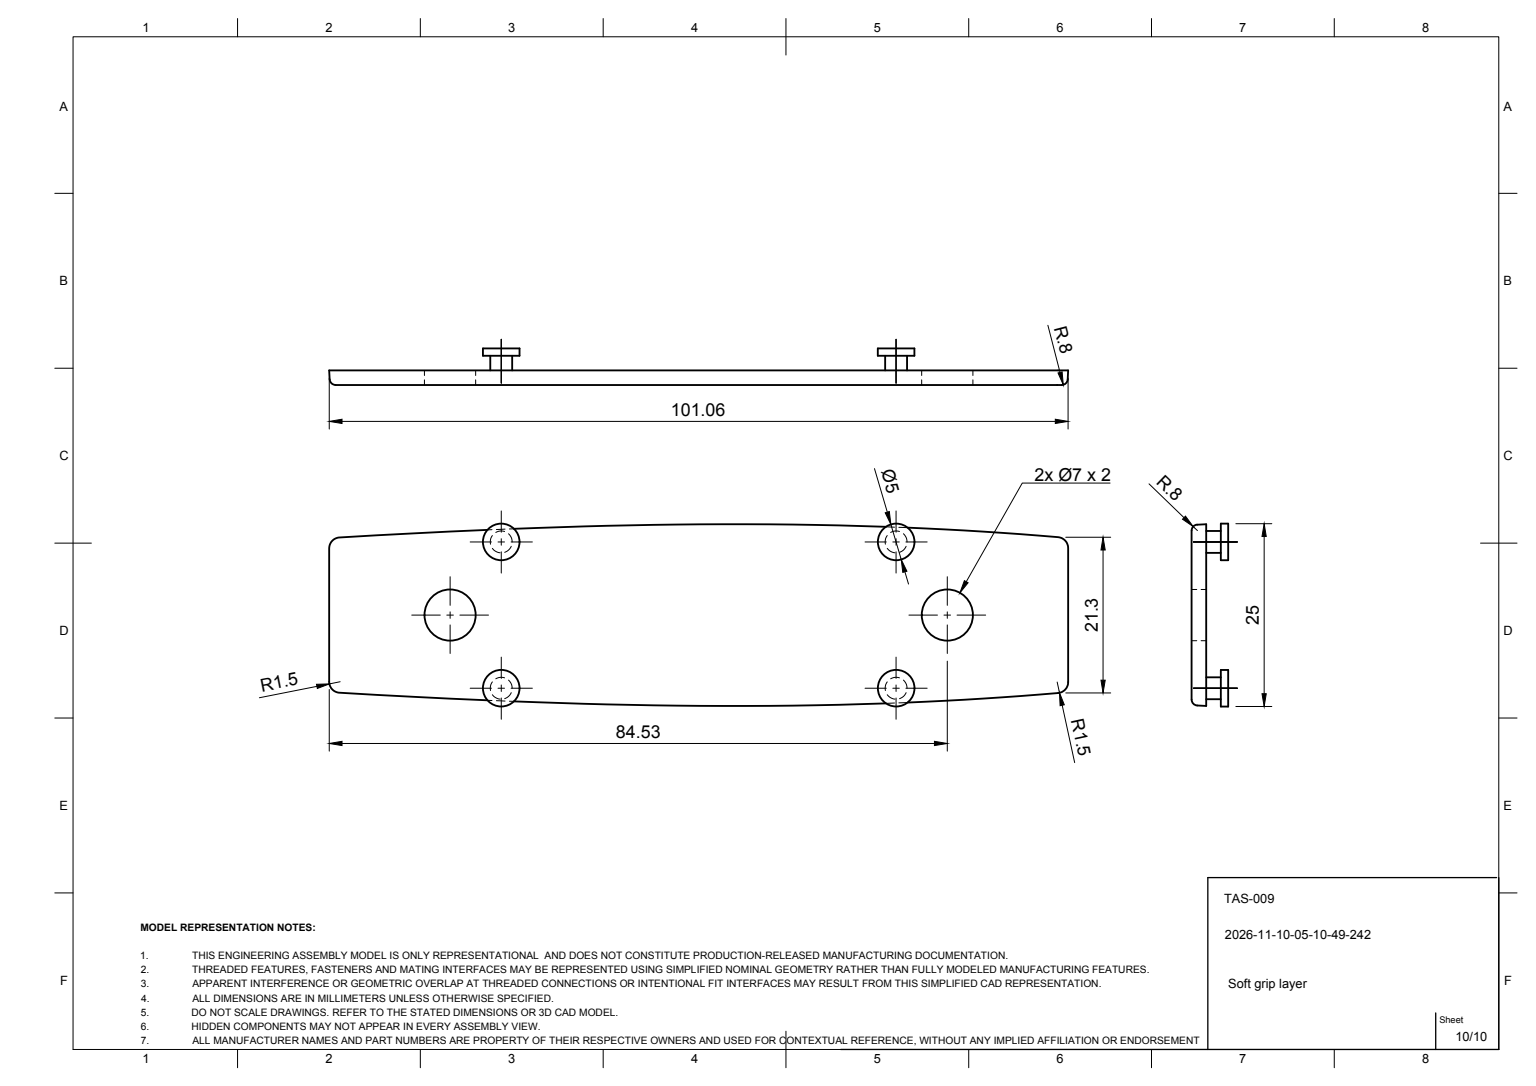
ISO-10303-21;
HEADER;
/* Generated by software containing ST-Developer
 * from STEP Tools, Inc. (www.steptools.com) 
 */

FILE_DESCRIPTION(
/* description */ (''),
/* implementation_level */ '2;1');

FILE_NAME(
/* name */ 'Soft grip layer.step',
/* time_stamp */ '2026-11-12T00:53:40-08:00',
/* author */ (''),
/* organization */ (''),
/* preprocessor_version */ 'ST-DEVELOPER v20.2',
/* originating_system */ 'Autodesk Translation Framework v15.17.0.0',
/* authorisation */ '');

FILE_SCHEMA (('AUTOMOTIVE_DESIGN { 1 0 10303 214 3 1 1 }'));
ENDSEC;

DATA;
#10=MECHANICAL_DESIGN_GEOMETRIC_PRESENTATION_REPRESENTATION('',(#579),#22129);
#160=B_SPLINE_SURFACE_WITH_KNOTS('',3,3,((#21557,#21558,#21559,#21560,#21561),
(#21562,#21563,#21564,#21565,#21566),(#21567,#21568,#21569,#21570,#21571),
(#21572,#21573,#21574,#21575,#21576),(#21577,#21578,#21579,#21580,#21581)),
 .UNSPECIFIED.,.F.,.F.,.F.,(4,1,4),(4,1,4),(0.,0.571428571428571,1.),(0.,
0.0453052401185593,0.105712226943305),.UNSPECIFIED.);
#161=B_SPLINE_SURFACE_WITH_KNOTS('',3,3,((#21604,#21605,#21606,#21607,#21608),
(#21609,#21610,#21611,#21612,#21613),(#21614,#21615,#21616,#21617,#21618),
(#21619,#21620,#21621,#21622,#21623),(#21624,#21625,#21626,#21627,#21628)),
 .UNSPECIFIED.,.F.,.F.,.F.,(4,1,4),(4,1,4),(0.,0.571428571428571,1.),(0.,
0.0453052401439183,0.105712227002476),.UNSPECIFIED.);
#162=B_SPLINE_SURFACE_WITH_KNOTS('',3,3,((#21642,#21643,#21644,#21645,#21646),
(#21647,#21648,#21649,#21650,#21651),(#21652,#21653,#21654,#21655,#21656),
(#21657,#21658,#21659,#21660,#21661),(#21662,#21663,#21664,#21665,#21666)),
 .UNSPECIFIED.,.F.,.F.,.F.,(4,1,4),(4,1,4),(0.,0.571428571428571,1.),(0.,
4.20509945658767,9.8118987320379),.UNSPECIFIED.);
#163=B_SPLINE_SURFACE_WITH_KNOTS('',3,3,((#21680,#21681,#21682,#21683,#21684),
(#21685,#21686,#21687,#21688,#21689),(#21690,#21691,#21692,#21693,#21694),
(#21695,#21696,#21697,#21698,#21699),(#21700,#21701,#21702,#21703,#21704)),
 .UNSPECIFIED.,.F.,.F.,.F.,(4,1,4),(4,1,4),(0.,0.571428571428571,1.),(0.,
0.0444882141544403,0.103805833027027),.UNSPECIFIED.);
#164=B_SPLINE_SURFACE_WITH_KNOTS('',3,3,((#21724,#21725,#21726,#21727,#21728),
(#21729,#21730,#21731,#21732,#21733),(#21734,#21735,#21736,#21737,#21738),
(#21739,#21740,#21741,#21742,#21743),(#21744,#21745,#21746,#21747,#21748)),
 .UNSPECIFIED.,.F.,.F.,.F.,(4,1,4),(4,1,4),(0.,0.571428571428571,1.),(2.06005858395869E-18,
0.0444882141931362,0.103805833117318),.UNSPECIFIED.);
#165=B_SPLINE_SURFACE_WITH_KNOTS('',3,3,((#21762,#21763,#21764,#21765,#21766),
(#21767,#21768,#21769,#21770,#21771),(#21772,#21773,#21774,#21775,#21776),
(#21777,#21778,#21779,#21780,#21781),(#21782,#21783,#21784,#21785,#21786)),
 .UNSPECIFIED.,.F.,.F.,.F.,(4,1,4),(4,1,4),(0.,0.571428571428571,1.),(0.,
4.20509909783593,9.81189789495051),.UNSPECIFIED.);
#166=B_SPLINE_SURFACE_WITH_KNOTS('',3,3,((#21809,#21810,#21811,#21812),
(#21813,#21814,#21815,#21816),(#21817,#21818,#21819,#21820),(#21821,#21822,
#21823,#21824),(#21825,#21826,#21827,#21828)),.UNSPECIFIED.,.F.,.F.,.F.,
(4,1,4),(4,4),(0.,0.571428571428571,1.),(-0.00268702576369722,0.125151053668407),
 .UNSPECIFIED.);
#167=B_SPLINE_SURFACE_WITH_KNOTS('',3,3,((#21862,#21863,#21864,#21865),
(#21866,#21867,#21868,#21869),(#21870,#21871,#21872,#21873),(#21874,#21875,
#21876,#21877)),.UNSPECIFIED.,.F.,.F.,.F.,(4,4),(4,4),(0.0135518988075539,
0.986045335056424),(0.,0.622596671418298),.UNSPECIFIED.);
#168=B_SPLINE_SURFACE_WITH_KNOTS('',3,3,((#21887,#21888,#21889,#21890),
(#21891,#21892,#21893,#21894),(#21895,#21896,#21897,#21898),(#21899,#21900,
#21901,#21902),(#21903,#21904,#21905,#21906)),.UNSPECIFIED.,.F.,.F.,.F.,
(4,1,4),(4,4),(0.,0.571428571428571,1.),(-0.00281084541253883,0.124959300034279),
 .UNSPECIFIED.);
#169=B_SPLINE_SURFACE_WITH_KNOTS('',3,3,((#21948,#21949,#21950,#21951),
(#21952,#21953,#21954,#21955),(#21956,#21957,#21958,#21959),(#21960,#21961,
#21962,#21963),(#21964,#21965,#21966,#21967)),.UNSPECIFIED.,.F.,.F.,.F.,
(4,1,4),(4,4),(0.,0.571428571428571,1.),(-0.00261432509268751,0.125151053668407),
 .UNSPECIFIED.);
#170=B_SPLINE_SURFACE_WITH_KNOTS('',3,3,((#22001,#22002,#22003,#22004),
(#22005,#22006,#22007,#22008),(#22009,#22010,#22011,#22012),(#22013,#22014,
#22015,#22016),(#22017,#22018,#22019,#22020)),.UNSPECIFIED.,.F.,.F.,.F.,
(4,1,4),(4,4),(0.,0.571428571428571,1.),(-0.00286362952972032,0.12495930003428),
 .UNSPECIFIED.);
#171=B_SPLINE_SURFACE_WITH_KNOTS('',3,3,((#22059,#22060,#22061,#22062),
(#22063,#22064,#22065,#22066),(#22067,#22068,#22069,#22070),(#22071,#22072,
#22073,#22074)),.UNSPECIFIED.,.F.,.F.,.F.,(4,4),(4,4),(0.0139546649435754,
0.986448101192446),(0.,0.622596671418299),.UNSPECIFIED.);
#528=B_SPLINE_CURVE_WITH_KNOTS('',3,(#21586,#21587,#21588,#21589,#21590),
 .UNSPECIFIED.,.F.,.F.,(4,1,4),(-0.105712226943305,-0.0453052401185593,
0.),.UNSPECIFIED.);
#529=B_SPLINE_CURVE_WITH_KNOTS('',3,(#21593,#21594,#21595,#21596,#21597),
 .UNSPECIFIED.,.F.,.F.,(4,1,4),(0.,0.0453052401185593,0.105712226943305),
 .UNSPECIFIED.);
#530=B_SPLINE_CURVE_WITH_KNOTS('',3,(#21632,#21633,#21634,#21635,#21636),
 .UNSPECIFIED.,.F.,.F.,(4,1,4),(-0.105712227002476,-0.0453052401439183,
0.),.UNSPECIFIED.);
#531=B_SPLINE_CURVE_WITH_KNOTS('',3,(#21637,#21638,#21639,#21640,#21641),
 .UNSPECIFIED.,.F.,.F.,(4,1,4),(0.,0.0453052401439183,0.105712227002476),
 .UNSPECIFIED.);
#532=B_SPLINE_CURVE_WITH_KNOTS('',3,(#21670,#21671,#21672,#21673,#21674),
 .UNSPECIFIED.,.F.,.F.,(4,1,4),(-9.8118987320379,-4.20509945658767,0.),
 .UNSPECIFIED.);
#533=B_SPLINE_CURVE_WITH_KNOTS('',3,(#21675,#21676,#21677,#21678,#21679),
 .UNSPECIFIED.,.F.,.F.,(4,1,4),(0.,4.20509945658767,9.8118987320379),
 .UNSPECIFIED.);
#534=B_SPLINE_CURVE_WITH_KNOTS('',3,(#21708,#21709,#21710,#21711,#21712),
 .UNSPECIFIED.,.F.,.F.,(4,1,4),(-0.103805833027027,-0.0444882141544403,
0.),.UNSPECIFIED.);
#535=B_SPLINE_CURVE_WITH_KNOTS('',3,(#21713,#21714,#21715,#21716,#21717),
 .UNSPECIFIED.,.F.,.F.,(4,1,4),(0.,0.0444882141544403,0.103805833027027),
 .UNSPECIFIED.);
#536=B_SPLINE_CURVE_WITH_KNOTS('',3,(#21752,#21753,#21754,#21755,#21756),
 .UNSPECIFIED.,.F.,.F.,(4,1,4),(-0.103805833117318,-0.0444882141931362,
-2.06005858395869E-18),.UNSPECIFIED.);
#537=B_SPLINE_CURVE_WITH_KNOTS('',3,(#21757,#21758,#21759,#21760,#21761),
 .UNSPECIFIED.,.F.,.F.,(4,1,4),(2.06005858395869E-18,0.0444882141931362,
0.103805833117318),.UNSPECIFIED.);
#538=B_SPLINE_CURVE_WITH_KNOTS('',3,(#21787,#21788,#21789,#21790,#21791),
 .UNSPECIFIED.,.F.,.F.,(4,1,4),(-9.81189789495051,-4.20509909783593,0.),
 .UNSPECIFIED.);
#539=B_SPLINE_CURVE_WITH_KNOTS('',3,(#21792,#21793,#21794,#21795,#21796),
 .UNSPECIFIED.,.F.,.F.,(4,1,4),(0.,4.20509909783593,9.81189789495051),
 .UNSPECIFIED.);
#540=B_SPLINE_CURVE_WITH_KNOTS('',3,(#21799,#21800,#21801,#21802),
 .UNSPECIFIED.,.F.,.F.,(4,4),(0.00062434729305816,0.125151053668407),
 .UNSPECIFIED.);
#541=B_SPLINE_CURVE_WITH_KNOTS('',3,(#21805,#21806,#21807,#21808),
 .UNSPECIFIED.,.F.,.F.,(4,4),(-0.125151053668407,-0.000624347293058304),
 .UNSPECIFIED.);
#542=B_SPLINE_CURVE_WITH_KNOTS('',3,(#21830,#21831,#21832,#21833),
 .UNSPECIFIED.,.F.,.F.,(4,4),(-0.124859357077656,3.91613824701764E-16),
 .UNSPECIFIED.);
#543=B_SPLINE_CURVE_WITH_KNOTS('',3,(#21834,#21835,#21836,#21837,#21838,
#21839,#21840,#21841,#21842,#21843,#21844,#21845,#21846,#21847,#21848,#21849,
#21850,#21851,#21852,#21853,#21854,#21855,#21856,#21857,#21858,#21859,#21860,
#21861),.UNSPECIFIED.,.F.,.F.,(4,3,3,3,3,3,3,3,3,4),(0.,0.032270992282214,
0.0586131010579366,0.0908535483049998,0.095660418056781,0.117090121226367,
0.149479430319939,0.17008966569926,0.202270498561131,0.223122165115773),
 .UNSPECIFIED.);
#544=B_SPLINE_CURVE_WITH_KNOTS('',3,(#21879,#21880,#21881,#21882),
 .UNSPECIFIED.,.F.,.F.,(4,4),(1.57426155444895E-16,0.124757292074316),
 .UNSPECIFIED.);
#545=B_SPLINE_CURVE_WITH_KNOTS('',3,(#21883,#21884,#21885,#21886),
 .UNSPECIFIED.,.F.,.F.,(4,4),(0.0135518988075539,0.986045335056425),
 .UNSPECIFIED.);
#546=B_SPLINE_CURVE_WITH_KNOTS('',3,(#21908,#21909,#21910,#21911),
 .UNSPECIFIED.,.F.,.F.,(4,4),(-0.124959300034279,-0.000432357919845506),
 .UNSPECIFIED.);
#547=B_SPLINE_CURVE_WITH_KNOTS('',3,(#21912,#21913,#21914,#21915,#21916,
#21917,#21918,#21919,#21920,#21921,#21922,#21923,#21924,#21925,#21926,#21927,
#21928,#21929,#21930,#21931,#21932,#21933,#21934,#21935,#21936,#21937,#21938,
#21939),.UNSPECIFIED.,.F.,.F.,(4,3,3,3,3,3,3,3,3,4),(0.,0.0322720371751271,
0.0586511315716134,0.0908889384397039,0.0974306796249642,0.117149930269381,
0.149553095257184,0.172178760978465,0.204364325027201,0.227238249760569),
 .UNSPECIFIED.);
#548=B_SPLINE_CURVE_WITH_KNOTS('',3,(#21943,#21944,#21945,#21946),
 .UNSPECIFIED.,.F.,.F.,(4,4),(0.000432357919845864,0.12495930003428),
 .UNSPECIFIED.);
#549=B_SPLINE_CURVE_WITH_KNOTS('',3,(#21969,#21970,#21971,#21972,#21973,
#21974,#21975,#21976,#21977,#21978,#21979,#21980,#21981,#21982,#21983,#21984,
#21985,#21986,#21987,#21988,#21989,#21990,#21991,#21992,#21993,#21994,#21995,
#21996),.UNSPECIFIED.,.F.,.F.,(4,3,3,3,3,3,3,3,3,4),(0.,0.0322770007607463,
0.0586509099358757,0.0908890592373503,0.0956758252683957,0.117149647541228,
0.149540928065794,0.17012301918783,0.202296660223156,0.2231241621482),
 .UNSPECIFIED.);
#550=B_SPLINE_CURVE_WITH_KNOTS('',3,(#21997,#21998,#21999,#22000),
 .UNSPECIFIED.,.F.,.F.,(4,4),(1.94722710178397E-16,0.124859357077656),
 .UNSPECIFIED.);
#551=B_SPLINE_CURVE_WITH_KNOTS('',3,(#22022,#22023,#22024,#22025),
 .UNSPECIFIED.,.F.,.F.,(4,4),(-0.124757292074297,-2.43294967505747E-16),
 .UNSPECIFIED.);
#552=B_SPLINE_CURVE_WITH_KNOTS('',3,(#22026,#22027,#22028,#22029,#22030,
#22031,#22032,#22033,#22034,#22035,#22036,#22037,#22038,#22039,#22040,#22041,
#22042,#22043,#22044,#22045,#22046,#22047,#22048,#22049,#22050,#22051,#22052,
#22053),.UNSPECIFIED.,.F.,.F.,(4,3,3,3,3,3,3,3,3,4),(0.,0.0322677829554273,
0.0586251784806003,0.0908644978360158,0.097419835848357,0.117108565494702,
0.149510109206483,0.172155480916619,0.204345933772222,0.227236831322489),
 .UNSPECIFIED.);
#553=B_SPLINE_CURVE_WITH_KNOTS('',3,(#22055,#22056,#22057,#22058),
 .UNSPECIFIED.,.F.,.F.,(4,4),(0.0139546649435756,0.986448101192446),
 .UNSPECIFIED.);
#561=SHAPE_REPRESENTATION_RELATIONSHIP('SRR','None',#22181,#570);
#570=ADVANCED_BREP_SHAPE_REPRESENTATION('',(#588),#22127);
#579=STYLED_ITEM('',(#22237),#588);
#588=MANIFOLD_SOLID_BREP('Body1',#8810);
#637=FACE_BOUND('',#1879,.T.);
#638=FACE_BOUND('',#1883,.T.);
#639=FACE_BOUND('',#1887,.T.);
#640=FACE_BOUND('',#1891,.T.);
#641=FACE_BOUND('',#1911,.T.);
#642=FACE_BOUND('',#1912,.T.);
#643=FACE_BOUND('',#1917,.T.);
#644=FACE_BOUND('',#1918,.T.);
#645=FACE_BOUND('',#1919,.T.);
#646=FACE_BOUND('',#1920,.T.);
#647=FACE_BOUND('',#1921,.T.);
#648=FACE_BOUND('',#1922,.T.);
#889=PLANE('',#9429);
#890=PLANE('',#9434);
#891=PLANE('',#9435);
#892=PLANE('',#9440);
#893=PLANE('',#9441);
#894=PLANE('',#9446);
#895=PLANE('',#9447);
#896=PLANE('',#9452);
#897=PLANE('',#9471);
#898=PLANE('',#9472);
#899=PLANE('',#9473);
#900=PLANE('',#9474);
#1346=FACE_OUTER_BOUND('',#1876,.T.);
#1347=FACE_OUTER_BOUND('',#1877,.T.);
#1348=FACE_OUTER_BOUND('',#1878,.T.);
#1349=FACE_OUTER_BOUND('',#1880,.T.);
#1350=FACE_OUTER_BOUND('',#1881,.T.);
#1351=FACE_OUTER_BOUND('',#1882,.T.);
#1352=FACE_OUTER_BOUND('',#1884,.T.);
#1353=FACE_OUTER_BOUND('',#1885,.T.);
#1354=FACE_OUTER_BOUND('',#1886,.T.);
#1355=FACE_OUTER_BOUND('',#1888,.T.);
#1356=FACE_OUTER_BOUND('',#1889,.T.);
#1357=FACE_OUTER_BOUND('',#1890,.T.);
#1358=FACE_OUTER_BOUND('',#1892,.T.);
#1359=FACE_OUTER_BOUND('',#1893,.T.);
#1360=FACE_OUTER_BOUND('',#1894,.T.);
#1361=FACE_OUTER_BOUND('',#1895,.T.);
#1362=FACE_OUTER_BOUND('',#1896,.T.);
#1363=FACE_OUTER_BOUND('',#1897,.T.);
#1364=FACE_OUTER_BOUND('',#1898,.T.);
#1365=FACE_OUTER_BOUND('',#1899,.T.);
#1366=FACE_OUTER_BOUND('',#1900,.T.);
#1367=FACE_OUTER_BOUND('',#1901,.T.);
#1368=FACE_OUTER_BOUND('',#1902,.T.);
#1369=FACE_OUTER_BOUND('',#1903,.T.);
#1370=FACE_OUTER_BOUND('',#1904,.T.);
#1371=FACE_OUTER_BOUND('',#1905,.T.);
#1372=FACE_OUTER_BOUND('',#1906,.T.);
#1373=FACE_OUTER_BOUND('',#1907,.T.);
#1374=FACE_OUTER_BOUND('',#1908,.T.);
#1375=FACE_OUTER_BOUND('',#1909,.T.);
#1376=FACE_OUTER_BOUND('',#1910,.T.);
#1377=FACE_OUTER_BOUND('',#1913,.T.);
#1378=FACE_OUTER_BOUND('',#1914,.T.);
#1379=FACE_OUTER_BOUND('',#1915,.T.);
#1380=FACE_OUTER_BOUND('',#1916,.T.);
#1381=FACE_OUTER_BOUND('',#1923,.T.);
#1876=EDGE_LOOP('',(#8034,#8035,#8036,#8037));
#1877=EDGE_LOOP('',(#8038,#8039,#8040,#8041));
#1878=EDGE_LOOP('',(#8042));
#1879=EDGE_LOOP('',(#8043));
#1880=EDGE_LOOP('',(#8044,#8045,#8046,#8047));
#1881=EDGE_LOOP('',(#8048));
#1882=EDGE_LOOP('',(#8049));
#1883=EDGE_LOOP('',(#8050));
#1884=EDGE_LOOP('',(#8051,#8052,#8053,#8054));
#1885=EDGE_LOOP('',(#8055));
#1886=EDGE_LOOP('',(#8056));
#1887=EDGE_LOOP('',(#8057));
#1888=EDGE_LOOP('',(#8058,#8059,#8060,#8061));
#1889=EDGE_LOOP('',(#8062));
#1890=EDGE_LOOP('',(#8063));
#1891=EDGE_LOOP('',(#8064));
#1892=EDGE_LOOP('',(#8065,#8066,#8067,#8068));
#1893=EDGE_LOOP('',(#8069));
#1894=EDGE_LOOP('',(#8070,#8071,#8072,#8073));
#1895=EDGE_LOOP('',(#8074,#8075,#8076,#8077));
#1896=EDGE_LOOP('',(#8078,#8079,#8080,#8081));
#1897=EDGE_LOOP('',(#8082,#8083,#8084,#8085));
#1898=EDGE_LOOP('',(#8086,#8087,#8088,#8089));
#1899=EDGE_LOOP('',(#8090,#8091,#8092,#8093));
#1900=EDGE_LOOP('',(#8094,#8095,#8096,#8097));
#1901=EDGE_LOOP('',(#8098,#8099,#8100,#8101));
#1902=EDGE_LOOP('',(#8102,#8103,#8104,#8105));
#1903=EDGE_LOOP('',(#8106,#8107,#8108,#8109));
#1904=EDGE_LOOP('',(#8110,#8111,#8112,#8113));
#1905=EDGE_LOOP('',(#8114,#8115,#8116,#8117));
#1906=EDGE_LOOP('',(#8118,#8119,#8120,#8121));
#1907=EDGE_LOOP('',(#8122,#8123,#8124,#8125));
#1908=EDGE_LOOP('',(#8126,#8127,#8128,#8129));
#1909=EDGE_LOOP('',(#8130,#8131,#8132,#8133));
#1910=EDGE_LOOP('',(#8134,#8135,#8136,#8137,#8138,#8139,#8140,#8141));
#1911=EDGE_LOOP('',(#8142));
#1912=EDGE_LOOP('',(#8143));
#1913=EDGE_LOOP('',(#8144,#8145,#8146,#8147));
#1914=EDGE_LOOP('',(#8148,#8149,#8150,#8151));
#1915=EDGE_LOOP('',(#8152,#8153,#8154,#8155));
#1916=EDGE_LOOP('',(#8156,#8157,#8158,#8159,#8160,#8161,#8162,#8163));
#1917=EDGE_LOOP('',(#8164));
#1918=EDGE_LOOP('',(#8165));
#1919=EDGE_LOOP('',(#8166));
#1920=EDGE_LOOP('',(#8167));
#1921=EDGE_LOOP('',(#8168));
#1922=EDGE_LOOP('',(#8169));
#1923=EDGE_LOOP('',(#8170,#8171,#8172,#8173));
#2642=LINE('',#21493,#3372);
#2643=LINE('',#21499,#3373);
#2644=LINE('',#21509,#3374);
#2645=LINE('',#21519,#3375);
#2646=LINE('',#21529,#3376);
#2647=LINE('',#21539,#3377);
#2648=LINE('',#21543,#3378);
#2649=LINE('',#21547,#3379);
#2650=LINE('',#21551,#3380);
#2651=LINE('',#21555,#3381);
#2652=LINE('',#21602,#3382);
#2653=LINE('',#21603,#3383);
#2654=LINE('',#21722,#3384);
#2655=LINE('',#21723,#3385);
#2656=LINE('',#21804,#3386);
#2657=LINE('',#21947,#3387);
#3372=VECTOR('',#11238,0.35);
#3373=VECTOR('',#11245,0.35);
#3374=VECTOR('',#11258,0.25);
#3375=VECTOR('',#11271,0.25);
#3376=VECTOR('',#11284,0.25);
#3377=VECTOR('',#11297,0.25);
#3378=VECTOR('',#11302,0.15);
#3379=VECTOR('',#11307,0.15);
#3380=VECTOR('',#11312,0.15);
#3381=VECTOR('',#11317,0.15);
#3382=VECTOR('',#11328,1.);
#3383=VECTOR('',#11329,1.);
#3384=VECTOR('',#11340,1.);
#3385=VECTOR('',#11341,1.);
#3386=VECTOR('',#11346,1.);
#3387=VECTOR('',#11351,1.);
#3516=CIRCLE('',#9424,0.35);
#3517=CIRCLE('',#9425,0.35);
#3518=CIRCLE('',#9427,0.35);
#3519=CIRCLE('',#9428,0.35);
#3520=CIRCLE('',#9430,0.25);
#3521=CIRCLE('',#9431,0.15);
#3522=CIRCLE('',#9433,0.25);
#3523=CIRCLE('',#9436,0.25);
#3524=CIRCLE('',#9437,0.15);
#3525=CIRCLE('',#9439,0.25);
#3526=CIRCLE('',#9442,0.25);
#3527=CIRCLE('',#9443,0.15);
#3528=CIRCLE('',#9445,0.25);
#3529=CIRCLE('',#9448,0.25);
#3530=CIRCLE('',#9449,0.15);
#3531=CIRCLE('',#9451,0.25);
#3532=CIRCLE('',#9454,0.15);
#3533=CIRCLE('',#9456,0.15);
#3534=CIRCLE('',#9458,0.15);
#3535=CIRCLE('',#9460,0.15);
#3536=CIRCLE('',#9461,0.0800000000000001);
#3537=CIRCLE('',#9462,0.0799999999999999);
#3538=CIRCLE('',#9464,0.0800000000000001);
#3539=CIRCLE('',#9465,0.0800000000000001);
#3540=CIRCLE('',#9466,0.0800000000000001);
#3541=CIRCLE('',#9467,0.0800000000000001);
#3542=CIRCLE('',#9469,0.0800000000000001);
#3543=CIRCLE('',#9470,0.0800000000000001);
#4328=VERTEX_POINT('',#21490);
#4329=VERTEX_POINT('',#21492);
#4330=VERTEX_POINT('',#21496);
#4331=VERTEX_POINT('',#21498);
#4332=VERTEX_POINT('',#21502);
#4333=VERTEX_POINT('',#21504);
#4334=VERTEX_POINT('',#21507);
#4335=VERTEX_POINT('',#21512);
#4336=VERTEX_POINT('',#21514);
#4337=VERTEX_POINT('',#21517);
#4338=VERTEX_POINT('',#21522);
#4339=VERTEX_POINT('',#21524);
#4340=VERTEX_POINT('',#21527);
#4341=VERTEX_POINT('',#21532);
#4342=VERTEX_POINT('',#21534);
#4343=VERTEX_POINT('',#21537);
#4344=VERTEX_POINT('',#21542);
#4345=VERTEX_POINT('',#21546);
#4346=VERTEX_POINT('',#21550);
#4347=VERTEX_POINT('',#21554);
#4348=VERTEX_POINT('',#21582);
#4349=VERTEX_POINT('',#21583);
#4350=VERTEX_POINT('',#21585);
#4351=VERTEX_POINT('',#21591);
#4352=VERTEX_POINT('',#21599);
#4353=VERTEX_POINT('',#21600);
#4354=VERTEX_POINT('',#21629);
#4355=VERTEX_POINT('',#21630);
#4356=VERTEX_POINT('',#21667);
#4357=VERTEX_POINT('',#21668);
#4358=VERTEX_POINT('',#21705);
#4359=VERTEX_POINT('',#21706);
#4360=VERTEX_POINT('',#21719);
#4361=VERTEX_POINT('',#21720);
#4362=VERTEX_POINT('',#21749);
#4363=VERTEX_POINT('',#21750);
#4364=VERTEX_POINT('',#21798);
#4365=VERTEX_POINT('',#21803);
#4366=VERTEX_POINT('',#21829);
#4367=VERTEX_POINT('',#21878);
#4368=VERTEX_POINT('',#21907);
#4369=VERTEX_POINT('',#21942);
#4370=VERTEX_POINT('',#21968);
#4371=VERTEX_POINT('',#22021);
#5570=EDGE_CURVE('',#4328,#4328,#3516,.T.);
#5571=EDGE_CURVE('',#4328,#4329,#2642,.T.);
#5572=EDGE_CURVE('',#4329,#4329,#3517,.T.);
#5573=EDGE_CURVE('',#4330,#4330,#3518,.T.);
#5574=EDGE_CURVE('',#4330,#4331,#2643,.T.);
#5575=EDGE_CURVE('',#4331,#4331,#3519,.T.);
#5576=EDGE_CURVE('',#4332,#4332,#3520,.T.);
#5577=EDGE_CURVE('',#4333,#4333,#3521,.T.);
#5578=EDGE_CURVE('',#4334,#4334,#3522,.T.);
#5579=EDGE_CURVE('',#4334,#4332,#2644,.T.);
#5580=EDGE_CURVE('',#4335,#4335,#3523,.T.);
#5581=EDGE_CURVE('',#4336,#4336,#3524,.T.);
#5582=EDGE_CURVE('',#4337,#4337,#3525,.T.);
#5583=EDGE_CURVE('',#4337,#4335,#2645,.T.);
#5584=EDGE_CURVE('',#4338,#4338,#3526,.T.);
#5585=EDGE_CURVE('',#4339,#4339,#3527,.T.);
#5586=EDGE_CURVE('',#4340,#4340,#3528,.T.);
#5587=EDGE_CURVE('',#4340,#4338,#2646,.T.);
#5588=EDGE_CURVE('',#4341,#4341,#3529,.T.);
#5589=EDGE_CURVE('',#4342,#4342,#3530,.T.);
#5590=EDGE_CURVE('',#4343,#4343,#3531,.T.);
#5591=EDGE_CURVE('',#4343,#4341,#2647,.T.);
#5592=EDGE_CURVE('',#4333,#4344,#2648,.T.);
#5593=EDGE_CURVE('',#4344,#4344,#3532,.T.);
#5594=EDGE_CURVE('',#4336,#4345,#2649,.T.);
#5595=EDGE_CURVE('',#4345,#4345,#3533,.T.);
#5596=EDGE_CURVE('',#4339,#4346,#2650,.T.);
#5597=EDGE_CURVE('',#4346,#4346,#3534,.T.);
#5598=EDGE_CURVE('',#4342,#4347,#2651,.T.);
#5599=EDGE_CURVE('',#4347,#4347,#3535,.T.);
#5600=EDGE_CURVE('',#4348,#4349,#3536,.T.);
#5601=EDGE_CURVE('',#4349,#4350,#528,.T.);
#5602=EDGE_CURVE('',#4350,#4351,#3537,.T.);
#5603=EDGE_CURVE('',#4351,#4348,#529,.T.);
#5604=EDGE_CURVE('',#4352,#4353,#3538,.T.);
#5605=EDGE_CURVE('',#4353,#4349,#2652,.T.);
#5606=EDGE_CURVE('',#4348,#4352,#2653,.T.);
#5607=EDGE_CURVE('',#4354,#4355,#3539,.T.);
#5608=EDGE_CURVE('',#4355,#4353,#530,.T.);
#5609=EDGE_CURVE('',#4352,#4354,#531,.T.);
#5610=EDGE_CURVE('',#4356,#4357,#3540,.T.);
#5611=EDGE_CURVE('',#4357,#4355,#532,.T.);
#5612=EDGE_CURVE('',#4354,#4356,#533,.T.);
#5613=EDGE_CURVE('',#4358,#4359,#3541,.T.);
#5614=EDGE_CURVE('',#4359,#4357,#534,.T.);
#5615=EDGE_CURVE('',#4356,#4358,#535,.T.);
#5616=EDGE_CURVE('',#4360,#4361,#3542,.T.);
#5617=EDGE_CURVE('',#4361,#4359,#2654,.T.);
#5618=EDGE_CURVE('',#4358,#4360,#2655,.T.);
#5619=EDGE_CURVE('',#4362,#4363,#3543,.T.);
#5620=EDGE_CURVE('',#4363,#4361,#536,.T.);
#5621=EDGE_CURVE('',#4360,#4362,#537,.T.);
#5622=EDGE_CURVE('',#4350,#4363,#538,.T.);
#5623=EDGE_CURVE('',#4362,#4351,#539,.T.);
#5624=EDGE_CURVE('',#4364,#4361,#540,.T.);
#5625=EDGE_CURVE('',#4365,#4364,#2656,.T.);
#5626=EDGE_CURVE('',#4359,#4365,#541,.T.);
#5627=EDGE_CURVE('',#4363,#4366,#542,.T.);
#5628=EDGE_CURVE('',#4366,#4364,#543,.T.);
#5629=EDGE_CURVE('',#4367,#4350,#544,.T.);
#5630=EDGE_CURVE('',#4366,#4367,#545,.T.);
#5631=EDGE_CURVE('',#4349,#4368,#546,.T.);
#5632=EDGE_CURVE('',#4368,#4367,#547,.T.);
#5633=EDGE_CURVE('',#4369,#4353,#548,.T.);
#5634=EDGE_CURVE('',#4368,#4369,#2657,.T.);
#5635=EDGE_CURVE('',#4365,#4370,#549,.T.);
#5636=EDGE_CURVE('',#4370,#4357,#550,.T.);
#5637=EDGE_CURVE('',#4355,#4371,#551,.T.);
#5638=EDGE_CURVE('',#4371,#4369,#552,.T.);
#5639=EDGE_CURVE('',#4371,#4370,#553,.T.);
#8034=ORIENTED_EDGE('',*,*,#5570,.F.);
#8035=ORIENTED_EDGE('',*,*,#5571,.T.);
#8036=ORIENTED_EDGE('',*,*,#5572,.F.);
#8037=ORIENTED_EDGE('',*,*,#5571,.F.);
#8038=ORIENTED_EDGE('',*,*,#5573,.F.);
#8039=ORIENTED_EDGE('',*,*,#5574,.T.);
#8040=ORIENTED_EDGE('',*,*,#5575,.F.);
#8041=ORIENTED_EDGE('',*,*,#5574,.F.);
#8042=ORIENTED_EDGE('',*,*,#5576,.T.);
#8043=ORIENTED_EDGE('',*,*,#5577,.T.);
#8044=ORIENTED_EDGE('',*,*,#5578,.F.);
#8045=ORIENTED_EDGE('',*,*,#5579,.T.);
#8046=ORIENTED_EDGE('',*,*,#5576,.F.);
#8047=ORIENTED_EDGE('',*,*,#5579,.F.);
#8048=ORIENTED_EDGE('',*,*,#5578,.T.);
#8049=ORIENTED_EDGE('',*,*,#5580,.T.);
#8050=ORIENTED_EDGE('',*,*,#5581,.T.);
#8051=ORIENTED_EDGE('',*,*,#5582,.F.);
#8052=ORIENTED_EDGE('',*,*,#5583,.T.);
#8053=ORIENTED_EDGE('',*,*,#5580,.F.);
#8054=ORIENTED_EDGE('',*,*,#5583,.F.);
#8055=ORIENTED_EDGE('',*,*,#5582,.T.);
#8056=ORIENTED_EDGE('',*,*,#5584,.T.);
#8057=ORIENTED_EDGE('',*,*,#5585,.T.);
#8058=ORIENTED_EDGE('',*,*,#5586,.F.);
#8059=ORIENTED_EDGE('',*,*,#5587,.T.);
#8060=ORIENTED_EDGE('',*,*,#5584,.F.);
#8061=ORIENTED_EDGE('',*,*,#5587,.F.);
#8062=ORIENTED_EDGE('',*,*,#5586,.T.);
#8063=ORIENTED_EDGE('',*,*,#5588,.T.);
#8064=ORIENTED_EDGE('',*,*,#5589,.T.);
#8065=ORIENTED_EDGE('',*,*,#5590,.F.);
#8066=ORIENTED_EDGE('',*,*,#5591,.T.);
#8067=ORIENTED_EDGE('',*,*,#5588,.F.);
#8068=ORIENTED_EDGE('',*,*,#5591,.F.);
#8069=ORIENTED_EDGE('',*,*,#5590,.T.);
#8070=ORIENTED_EDGE('',*,*,#5577,.F.);
#8071=ORIENTED_EDGE('',*,*,#5592,.T.);
#8072=ORIENTED_EDGE('',*,*,#5593,.F.);
#8073=ORIENTED_EDGE('',*,*,#5592,.F.);
#8074=ORIENTED_EDGE('',*,*,#5581,.F.);
#8075=ORIENTED_EDGE('',*,*,#5594,.T.);
#8076=ORIENTED_EDGE('',*,*,#5595,.F.);
#8077=ORIENTED_EDGE('',*,*,#5594,.F.);
#8078=ORIENTED_EDGE('',*,*,#5585,.F.);
#8079=ORIENTED_EDGE('',*,*,#5596,.T.);
#8080=ORIENTED_EDGE('',*,*,#5597,.F.);
#8081=ORIENTED_EDGE('',*,*,#5596,.F.);
#8082=ORIENTED_EDGE('',*,*,#5589,.F.);
#8083=ORIENTED_EDGE('',*,*,#5598,.T.);
#8084=ORIENTED_EDGE('',*,*,#5599,.F.);
#8085=ORIENTED_EDGE('',*,*,#5598,.F.);
#8086=ORIENTED_EDGE('',*,*,#5600,.T.);
#8087=ORIENTED_EDGE('',*,*,#5601,.T.);
#8088=ORIENTED_EDGE('',*,*,#5602,.T.);
#8089=ORIENTED_EDGE('',*,*,#5603,.T.);
#8090=ORIENTED_EDGE('',*,*,#5604,.T.);
#8091=ORIENTED_EDGE('',*,*,#5605,.T.);
#8092=ORIENTED_EDGE('',*,*,#5600,.F.);
#8093=ORIENTED_EDGE('',*,*,#5606,.T.);
#8094=ORIENTED_EDGE('',*,*,#5607,.T.);
#8095=ORIENTED_EDGE('',*,*,#5608,.T.);
#8096=ORIENTED_EDGE('',*,*,#5604,.F.);
#8097=ORIENTED_EDGE('',*,*,#5609,.T.);
#8098=ORIENTED_EDGE('',*,*,#5610,.T.);
#8099=ORIENTED_EDGE('',*,*,#5611,.T.);
#8100=ORIENTED_EDGE('',*,*,#5607,.F.);
#8101=ORIENTED_EDGE('',*,*,#5612,.T.);
#8102=ORIENTED_EDGE('',*,*,#5613,.T.);
#8103=ORIENTED_EDGE('',*,*,#5614,.T.);
#8104=ORIENTED_EDGE('',*,*,#5610,.F.);
#8105=ORIENTED_EDGE('',*,*,#5615,.T.);
#8106=ORIENTED_EDGE('',*,*,#5616,.T.);
#8107=ORIENTED_EDGE('',*,*,#5617,.T.);
#8108=ORIENTED_EDGE('',*,*,#5613,.F.);
#8109=ORIENTED_EDGE('',*,*,#5618,.T.);
#8110=ORIENTED_EDGE('',*,*,#5619,.T.);
#8111=ORIENTED_EDGE('',*,*,#5620,.T.);
#8112=ORIENTED_EDGE('',*,*,#5616,.F.);
#8113=ORIENTED_EDGE('',*,*,#5621,.T.);
#8114=ORIENTED_EDGE('',*,*,#5602,.F.);
#8115=ORIENTED_EDGE('',*,*,#5622,.T.);
#8116=ORIENTED_EDGE('',*,*,#5619,.F.);
#8117=ORIENTED_EDGE('',*,*,#5623,.T.);
#8118=ORIENTED_EDGE('',*,*,#5617,.F.);
#8119=ORIENTED_EDGE('',*,*,#5624,.F.);
#8120=ORIENTED_EDGE('',*,*,#5625,.F.);
#8121=ORIENTED_EDGE('',*,*,#5626,.F.);
#8122=ORIENTED_EDGE('',*,*,#5620,.F.);
#8123=ORIENTED_EDGE('',*,*,#5627,.T.);
#8124=ORIENTED_EDGE('',*,*,#5628,.T.);
#8125=ORIENTED_EDGE('',*,*,#5624,.T.);
#8126=ORIENTED_EDGE('',*,*,#5622,.F.);
#8127=ORIENTED_EDGE('',*,*,#5629,.F.);
#8128=ORIENTED_EDGE('',*,*,#5630,.F.);
#8129=ORIENTED_EDGE('',*,*,#5627,.F.);
#8130=ORIENTED_EDGE('',*,*,#5601,.F.);
#8131=ORIENTED_EDGE('',*,*,#5631,.T.);
#8132=ORIENTED_EDGE('',*,*,#5632,.T.);
#8133=ORIENTED_EDGE('',*,*,#5629,.T.);
#8134=ORIENTED_EDGE('',*,*,#5603,.F.);
#8135=ORIENTED_EDGE('',*,*,#5623,.F.);
#8136=ORIENTED_EDGE('',*,*,#5621,.F.);
#8137=ORIENTED_EDGE('',*,*,#5618,.F.);
#8138=ORIENTED_EDGE('',*,*,#5615,.F.);
#8139=ORIENTED_EDGE('',*,*,#5612,.F.);
#8140=ORIENTED_EDGE('',*,*,#5609,.F.);
#8141=ORIENTED_EDGE('',*,*,#5606,.F.);
#8142=ORIENTED_EDGE('',*,*,#5570,.T.);
#8143=ORIENTED_EDGE('',*,*,#5573,.T.);
#8144=ORIENTED_EDGE('',*,*,#5605,.F.);
#8145=ORIENTED_EDGE('',*,*,#5633,.F.);
#8146=ORIENTED_EDGE('',*,*,#5634,.F.);
#8147=ORIENTED_EDGE('',*,*,#5631,.F.);
#8148=ORIENTED_EDGE('',*,*,#5614,.F.);
#8149=ORIENTED_EDGE('',*,*,#5626,.T.);
#8150=ORIENTED_EDGE('',*,*,#5635,.T.);
#8151=ORIENTED_EDGE('',*,*,#5636,.T.);
#8152=ORIENTED_EDGE('',*,*,#5608,.F.);
#8153=ORIENTED_EDGE('',*,*,#5637,.T.);
#8154=ORIENTED_EDGE('',*,*,#5638,.T.);
#8155=ORIENTED_EDGE('',*,*,#5633,.T.);
#8156=ORIENTED_EDGE('',*,*,#5632,.F.);
#8157=ORIENTED_EDGE('',*,*,#5634,.T.);
#8158=ORIENTED_EDGE('',*,*,#5638,.F.);
#8159=ORIENTED_EDGE('',*,*,#5639,.T.);
#8160=ORIENTED_EDGE('',*,*,#5635,.F.);
#8161=ORIENTED_EDGE('',*,*,#5625,.T.);
#8162=ORIENTED_EDGE('',*,*,#5628,.F.);
#8163=ORIENTED_EDGE('',*,*,#5630,.T.);
#8164=ORIENTED_EDGE('',*,*,#5572,.T.);
#8165=ORIENTED_EDGE('',*,*,#5575,.T.);
#8166=ORIENTED_EDGE('',*,*,#5593,.T.);
#8167=ORIENTED_EDGE('',*,*,#5595,.T.);
#8168=ORIENTED_EDGE('',*,*,#5597,.T.);
#8169=ORIENTED_EDGE('',*,*,#5599,.T.);
#8170=ORIENTED_EDGE('',*,*,#5611,.F.);
#8171=ORIENTED_EDGE('',*,*,#5636,.F.);
#8172=ORIENTED_EDGE('',*,*,#5639,.F.);
#8173=ORIENTED_EDGE('',*,*,#5637,.F.);
#8306=CYLINDRICAL_SURFACE('',#9423,0.35);
#8307=CYLINDRICAL_SURFACE('',#9426,0.35);
#8308=CYLINDRICAL_SURFACE('',#9432,0.25);
#8309=CYLINDRICAL_SURFACE('',#9438,0.25);
#8310=CYLINDRICAL_SURFACE('',#9444,0.25);
#8311=CYLINDRICAL_SURFACE('',#9450,0.25);
#8312=CYLINDRICAL_SURFACE('',#9453,0.15);
#8313=CYLINDRICAL_SURFACE('',#9455,0.15);
#8314=CYLINDRICAL_SURFACE('',#9457,0.15);
#8315=CYLINDRICAL_SURFACE('',#9459,0.15);
#8316=CYLINDRICAL_SURFACE('',#9463,0.08);
#8317=CYLINDRICAL_SURFACE('',#9468,0.08);
#8763=ADVANCED_FACE('',(#1346),#8306,.F.);
#8764=ADVANCED_FACE('',(#1347),#8307,.F.);
#8765=ADVANCED_FACE('',(#1348,#637),#889,.T.);
#8766=ADVANCED_FACE('',(#1349),#8308,.T.);
#8767=ADVANCED_FACE('',(#1350),#890,.F.);
#8768=ADVANCED_FACE('',(#1351,#638),#891,.T.);
#8769=ADVANCED_FACE('',(#1352),#8309,.T.);
#8770=ADVANCED_FACE('',(#1353),#892,.F.);
#8771=ADVANCED_FACE('',(#1354,#639),#893,.T.);
#8772=ADVANCED_FACE('',(#1355),#8310,.T.);
#8773=ADVANCED_FACE('',(#1356),#894,.F.);
#8774=ADVANCED_FACE('',(#1357,#640),#895,.T.);
#8775=ADVANCED_FACE('',(#1358),#8311,.T.);
#8776=ADVANCED_FACE('',(#1359),#896,.F.);
#8777=ADVANCED_FACE('',(#1360),#8312,.T.);
#8778=ADVANCED_FACE('',(#1361),#8313,.T.);
#8779=ADVANCED_FACE('',(#1362),#8314,.T.);
#8780=ADVANCED_FACE('',(#1363),#8315,.T.);
#8781=ADVANCED_FACE('',(#1364),#160,.F.);
#8782=ADVANCED_FACE('',(#1365),#8316,.T.);
#8783=ADVANCED_FACE('',(#1366),#161,.F.);
#8784=ADVANCED_FACE('',(#1367),#162,.F.);
#8785=ADVANCED_FACE('',(#1368),#163,.F.);
#8786=ADVANCED_FACE('',(#1369),#8317,.T.);
#8787=ADVANCED_FACE('',(#1370),#164,.F.);
#8788=ADVANCED_FACE('',(#1371),#165,.F.);
#8789=ADVANCED_FACE('',(#1372),#897,.F.);
#8790=ADVANCED_FACE('',(#1373),#166,.F.);
#8791=ADVANCED_FACE('',(#1374),#167,.F.);
#8792=ADVANCED_FACE('',(#1375),#168,.F.);
#8793=ADVANCED_FACE('',(#1376,#641,#642),#898,.T.);
#8794=ADVANCED_FACE('',(#1377),#899,.F.);
#8795=ADVANCED_FACE('',(#1378),#169,.F.);
#8796=ADVANCED_FACE('',(#1379),#170,.F.);
#8797=ADVANCED_FACE('',(#1380,#643,#644,#645,#646,#647,#648),#900,.F.);
#8798=ADVANCED_FACE('',(#1381),#171,.F.);
#8810=CLOSED_SHELL('',(#8763,#8764,#8765,#8766,#8767,#8768,#8769,#8770,
#8771,#8772,#8773,#8774,#8775,#8776,#8777,#8778,#8779,#8780,#8781,#8782,
#8783,#8784,#8785,#8786,#8787,#8788,#8789,#8790,#8791,#8792,#8793,#8794,
#8795,#8796,#8797,#8798));
#9422=AXIS2_PLACEMENT_3D('',#21488,#11232,#11233);
#9423=AXIS2_PLACEMENT_3D('',#21489,#11234,#11235);
#9424=AXIS2_PLACEMENT_3D('',#21491,#11236,#11237);
#9425=AXIS2_PLACEMENT_3D('',#21494,#11239,#11240);
#9426=AXIS2_PLACEMENT_3D('',#21495,#11241,#11242);
#9427=AXIS2_PLACEMENT_3D('',#21497,#11243,#11244);
#9428=AXIS2_PLACEMENT_3D('',#21500,#11246,#11247);
#9429=AXIS2_PLACEMENT_3D('',#21501,#11248,#11249);
#9430=AXIS2_PLACEMENT_3D('',#21503,#11250,#11251);
#9431=AXIS2_PLACEMENT_3D('',#21505,#11252,#11253);
#9432=AXIS2_PLACEMENT_3D('',#21506,#11254,#11255);
#9433=AXIS2_PLACEMENT_3D('',#21508,#11256,#11257);
#9434=AXIS2_PLACEMENT_3D('',#21510,#11259,#11260);
#9435=AXIS2_PLACEMENT_3D('',#21511,#11261,#11262);
#9436=AXIS2_PLACEMENT_3D('',#21513,#11263,#11264);
#9437=AXIS2_PLACEMENT_3D('',#21515,#11265,#11266);
#9438=AXIS2_PLACEMENT_3D('',#21516,#11267,#11268);
#9439=AXIS2_PLACEMENT_3D('',#21518,#11269,#11270);
#9440=AXIS2_PLACEMENT_3D('',#21520,#11272,#11273);
#9441=AXIS2_PLACEMENT_3D('',#21521,#11274,#11275);
#9442=AXIS2_PLACEMENT_3D('',#21523,#11276,#11277);
#9443=AXIS2_PLACEMENT_3D('',#21525,#11278,#11279);
#9444=AXIS2_PLACEMENT_3D('',#21526,#11280,#11281);
#9445=AXIS2_PLACEMENT_3D('',#21528,#11282,#11283);
#9446=AXIS2_PLACEMENT_3D('',#21530,#11285,#11286);
#9447=AXIS2_PLACEMENT_3D('',#21531,#11287,#11288);
#9448=AXIS2_PLACEMENT_3D('',#21533,#11289,#11290);
#9449=AXIS2_PLACEMENT_3D('',#21535,#11291,#11292);
#9450=AXIS2_PLACEMENT_3D('',#21536,#11293,#11294);
#9451=AXIS2_PLACEMENT_3D('',#21538,#11295,#11296);
#9452=AXIS2_PLACEMENT_3D('',#21540,#11298,#11299);
#9453=AXIS2_PLACEMENT_3D('',#21541,#11300,#11301);
#9454=AXIS2_PLACEMENT_3D('',#21544,#11303,#11304);
#9455=AXIS2_PLACEMENT_3D('',#21545,#11305,#11306);
#9456=AXIS2_PLACEMENT_3D('',#21548,#11308,#11309);
#9457=AXIS2_PLACEMENT_3D('',#21549,#11310,#11311);
#9458=AXIS2_PLACEMENT_3D('',#21552,#11313,#11314);
#9459=AXIS2_PLACEMENT_3D('',#21553,#11315,#11316);
#9460=AXIS2_PLACEMENT_3D('',#21556,#11318,#11319);
#9461=AXIS2_PLACEMENT_3D('',#21584,#11320,#11321);
#9462=AXIS2_PLACEMENT_3D('',#21592,#11322,#11323);
#9463=AXIS2_PLACEMENT_3D('',#21598,#11324,#11325);
#9464=AXIS2_PLACEMENT_3D('',#21601,#11326,#11327);
#9465=AXIS2_PLACEMENT_3D('',#21631,#11330,#11331);
#9466=AXIS2_PLACEMENT_3D('',#21669,#11332,#11333);
#9467=AXIS2_PLACEMENT_3D('',#21707,#11334,#11335);
#9468=AXIS2_PLACEMENT_3D('',#21718,#11336,#11337);
#9469=AXIS2_PLACEMENT_3D('',#21721,#11338,#11339);
#9470=AXIS2_PLACEMENT_3D('',#21751,#11342,#11343);
#9471=AXIS2_PLACEMENT_3D('',#21797,#11344,#11345);
#9472=AXIS2_PLACEMENT_3D('',#21940,#11347,#11348);
#9473=AXIS2_PLACEMENT_3D('',#21941,#11349,#11350);
#9474=AXIS2_PLACEMENT_3D('',#22054,#11352,#11353);
#11232=DIRECTION('axis',(0.,0.,1.));
#11233=DIRECTION('refdir',(1.,0.,0.));
#11234=DIRECTION('center_axis',(0.,0.,-1.));
#11235=DIRECTION('ref_axis',(1.,0.,0.));
#11236=DIRECTION('center_axis',(1.16928610669829E-31,-5.97538301968883E-32,
-1.));
#11237=DIRECTION('ref_axis',(1.,0.,0.));
#11238=DIRECTION('',(0.,0.,-1.));
#11239=DIRECTION('center_axis',(-6.45616000593692E-32,-1.81182428107391E-19,
1.));
#11240=DIRECTION('ref_axis',(1.,0.,0.));
#11241=DIRECTION('center_axis',(0.,0.,-1.));
#11242=DIRECTION('ref_axis',(1.,0.,0.));
#11243=DIRECTION('center_axis',(1.16928610669829E-31,-5.97538301968883E-32,
-1.));
#11244=DIRECTION('ref_axis',(1.,0.,0.));
#11245=DIRECTION('',(0.,0.,-1.));
#11246=DIRECTION('center_axis',(-6.45616000593692E-32,-1.81182428107391E-19,
1.));
#11247=DIRECTION('ref_axis',(1.,0.,0.));
#11248=DIRECTION('center_axis',(0.,0.,1.));
#11249=DIRECTION('ref_axis',(1.,0.,0.));
#11250=DIRECTION('center_axis',(0.,0.,1.));
#11251=DIRECTION('ref_axis',(1.,0.,0.));
#11252=DIRECTION('center_axis',(0.,0.,-1.));
#11253=DIRECTION('ref_axis',(1.,0.,0.));
#11254=DIRECTION('center_axis',(0.,0.,-1.));
#11255=DIRECTION('ref_axis',(1.,0.,0.));
#11256=DIRECTION('center_axis',(0.,0.,-1.));
#11257=DIRECTION('ref_axis',(1.,0.,0.));
#11258=DIRECTION('',(0.,0.,1.));
#11259=DIRECTION('center_axis',(0.,0.,1.));
#11260=DIRECTION('ref_axis',(1.,0.,0.));
#11261=DIRECTION('center_axis',(0.,0.,1.));
#11262=DIRECTION('ref_axis',(1.,0.,0.));
#11263=DIRECTION('center_axis',(0.,0.,1.));
#11264=DIRECTION('ref_axis',(1.,0.,0.));
#11265=DIRECTION('center_axis',(0.,0.,-1.));
#11266=DIRECTION('ref_axis',(1.,0.,0.));
#11267=DIRECTION('center_axis',(0.,0.,-1.));
#11268=DIRECTION('ref_axis',(1.,0.,0.));
#11269=DIRECTION('center_axis',(0.,0.,-1.));
#11270=DIRECTION('ref_axis',(1.,0.,0.));
#11271=DIRECTION('',(0.,0.,1.));
#11272=DIRECTION('center_axis',(0.,0.,1.));
#11273=DIRECTION('ref_axis',(1.,0.,0.));
#11274=DIRECTION('center_axis',(0.,0.,1.));
#11275=DIRECTION('ref_axis',(1.,0.,0.));
#11276=DIRECTION('center_axis',(0.,0.,1.));
#11277=DIRECTION('ref_axis',(1.,0.,0.));
#11278=DIRECTION('center_axis',(0.,0.,-1.));
#11279=DIRECTION('ref_axis',(1.,0.,0.));
#11280=DIRECTION('center_axis',(0.,0.,-1.));
#11281=DIRECTION('ref_axis',(1.,0.,0.));
#11282=DIRECTION('center_axis',(0.,0.,-1.));
#11283=DIRECTION('ref_axis',(1.,0.,0.));
#11284=DIRECTION('',(0.,0.,1.));
#11285=DIRECTION('center_axis',(0.,0.,1.));
#11286=DIRECTION('ref_axis',(1.,0.,0.));
#11287=DIRECTION('center_axis',(0.,0.,1.));
#11288=DIRECTION('ref_axis',(1.,0.,0.));
#11289=DIRECTION('center_axis',(0.,0.,1.));
#11290=DIRECTION('ref_axis',(1.,0.,0.));
#11291=DIRECTION('center_axis',(0.,0.,-1.));
#11292=DIRECTION('ref_axis',(1.,0.,0.));
#11293=DIRECTION('center_axis',(0.,0.,-1.));
#11294=DIRECTION('ref_axis',(1.,0.,0.));
#11295=DIRECTION('center_axis',(0.,0.,-1.));
#11296=DIRECTION('ref_axis',(1.,0.,0.));
#11297=DIRECTION('',(0.,0.,1.));
#11298=DIRECTION('center_axis',(0.,0.,1.));
#11299=DIRECTION('ref_axis',(1.,0.,0.));
#11300=DIRECTION('center_axis',(0.,0.,-1.));
#11301=DIRECTION('ref_axis',(1.,0.,0.));
#11302=DIRECTION('',(0.,0.,1.));
#11303=DIRECTION('center_axis',(-6.45616000593692E-32,-1.81182428107391E-19,
1.));
#11304=DIRECTION('ref_axis',(1.,0.,0.));
#11305=DIRECTION('center_axis',(0.,0.,-1.));
#11306=DIRECTION('ref_axis',(1.,0.,0.));
#11307=DIRECTION('',(0.,0.,1.));
#11308=DIRECTION('center_axis',(-6.45616000593692E-32,-1.81182428107391E-19,
1.));
#11309=DIRECTION('ref_axis',(1.,0.,0.));
#11310=DIRECTION('center_axis',(0.,0.,-1.));
#11311=DIRECTION('ref_axis',(1.,0.,0.));
#11312=DIRECTION('',(0.,0.,1.));
#11313=DIRECTION('center_axis',(-6.45616000593692E-32,-1.81182428107391E-19,
1.));
#11314=DIRECTION('ref_axis',(1.,0.,0.));
#11315=DIRECTION('center_axis',(0.,0.,-1.));
#11316=DIRECTION('ref_axis',(1.,0.,0.));
#11317=DIRECTION('',(0.,0.,1.));
#11318=DIRECTION('center_axis',(-6.45616000593692E-32,-1.81182428107391E-19,
1.));
#11319=DIRECTION('ref_axis',(1.,0.,0.));
#11320=DIRECTION('center_axis',(0.,1.,0.));
#11321=DIRECTION('ref_axis',(0.,0.,1.));
#11322=DIRECTION('center_axis',(0.998287351281347,-0.0585009766728139,0.));
#11323=DIRECTION('ref_axis',(0.0584117362954384,0.996764512774636,0.0552139034672828));
#11324=DIRECTION('center_axis',(-3.13156554427463E-33,-1.,5.97538301968883E-32));
#11325=DIRECTION('ref_axis',(0.688354575693766,0.,0.725374371012276));
#11326=DIRECTION('center_axis',(1.38968329343724E-15,1.,0.));
#11327=DIRECTION('ref_axis',(0.,0.,1.));
#11328=DIRECTION('',(3.13156554427463E-33,1.,-5.97538301968883E-32));
#11329=DIRECTION('',(-3.13156554427463E-33,-1.,5.97538301968883E-32));
#11330=DIRECTION('center_axis',(0.998287351281345,0.0585009766728351,0.));
#11331=DIRECTION('ref_axis',(0.,0.,1.));
#11332=DIRECTION('center_axis',(0.996325437245183,-0.0856482521607663,0.));
#11333=DIRECTION('ref_axis',(0.,0.,1.));
#11334=DIRECTION('center_axis',(-1.38968329343725E-15,-1.,-6.75000545323542E-30));
#11335=DIRECTION('ref_axis',(-4.85722573273506E-15,0.,1.));
#11336=DIRECTION('center_axis',(-3.13156554427485E-33,1.,-5.97538301968883E-32));
#11337=DIRECTION('ref_axis',(-0.688354575693752,0.,0.72537437101229));
#11338=DIRECTION('center_axis',(1.38968329343726E-15,-1.,0.));
#11339=DIRECTION('ref_axis',(0.,0.,1.));
#11340=DIRECTION('',(3.13156554427485E-33,-1.,5.97538301968883E-32));
#11341=DIRECTION('',(-3.13156554427485E-33,1.,-5.97538301968883E-32));
#11342=DIRECTION('center_axis',(-0.996325437245184,-0.0856482521607654,
-4.83937755196581E-15));
#11343=DIRECTION('ref_axis',(-4.85722573273506E-15,0.,1.));
#11344=DIRECTION('center_axis',(0.998629534754574,0.,-0.0523359562429439));
#11345=DIRECTION('ref_axis',(-0.0523359562429439,0.,-0.998629534754574));
#11346=DIRECTION('',(0.,1.,0.));
#11347=DIRECTION('center_axis',(-1.16928610669829E-31,5.97538301968883E-32,
1.));
#11348=DIRECTION('ref_axis',(1.,0.,1.16928610669829E-31));
#11349=DIRECTION('center_axis',(-0.998629534754574,0.,-0.0523359562429402));
#11350=DIRECTION('ref_axis',(-0.0523359562429402,0.,0.998629534754574));
#11351=DIRECTION('',(0.,-1.,0.));
#11352=DIRECTION('center_axis',(-6.45616000593692E-32,-1.81182428107391E-19,
1.));
#11353=DIRECTION('ref_axis',(1.,0.,6.45616000593692E-32));
#21488=CARTESIAN_POINT('',(0.,0.,0.));
#21489=CARTESIAN_POINT('Origin',(2.,0.,1.));
#21490=CARTESIAN_POINT('',(1.65,4.28626379701574E-17,1.1));
#21491=CARTESIAN_POINT('Origin',(2.,0.,1.1));
#21492=CARTESIAN_POINT('',(1.65,4.28626379701574E-17,0.9));
#21493=CARTESIAN_POINT('',(1.65,4.28626379701574E-17,1.));
#21494=CARTESIAN_POINT('Origin',(2.,0.,0.9));
#21495=CARTESIAN_POINT('Origin',(8.8,0.,1.));
#21496=CARTESIAN_POINT('',(8.45,4.28626379701574E-17,1.1));
#21497=CARTESIAN_POINT('Origin',(8.8,0.,1.1));
#21498=CARTESIAN_POINT('',(8.45,4.28626379701574E-17,0.9));
#21499=CARTESIAN_POINT('',(8.45,4.28626379701574E-17,1.));
#21500=CARTESIAN_POINT('Origin',(8.8,0.,0.9));
#21501=CARTESIAN_POINT('Origin',(8.1,1.,0.7));
#21502=CARTESIAN_POINT('',(7.85,1.,0.7));
#21503=CARTESIAN_POINT('Origin',(8.1,1.,0.7));
#21504=CARTESIAN_POINT('',(7.95,1.,0.7));
#21505=CARTESIAN_POINT('Origin',(8.1,1.,0.7));
#21506=CARTESIAN_POINT('Origin',(8.1,1.,0.7));
#21507=CARTESIAN_POINT('',(7.85,1.,0.6));
#21508=CARTESIAN_POINT('Origin',(8.1,1.,0.6));
#21509=CARTESIAN_POINT('',(7.85,1.,0.7));
#21510=CARTESIAN_POINT('Origin',(8.1,1.,0.6));
#21511=CARTESIAN_POINT('Origin',(2.7,-1.,0.7));
#21512=CARTESIAN_POINT('',(2.45,-1.,0.7));
#21513=CARTESIAN_POINT('Origin',(2.7,-1.,0.7));
#21514=CARTESIAN_POINT('',(2.55,-1.,0.7));
#21515=CARTESIAN_POINT('Origin',(2.7,-1.,0.7));
#21516=CARTESIAN_POINT('Origin',(2.7,-1.,0.7));
#21517=CARTESIAN_POINT('',(2.45,-1.,0.6));
#21518=CARTESIAN_POINT('Origin',(2.7,-1.,0.6));
#21519=CARTESIAN_POINT('',(2.45,-1.,0.7));
#21520=CARTESIAN_POINT('Origin',(2.7,-1.,0.6));
#21521=CARTESIAN_POINT('Origin',(2.7,1.,0.7));
#21522=CARTESIAN_POINT('',(2.45,1.,0.7));
#21523=CARTESIAN_POINT('Origin',(2.7,1.,0.7));
#21524=CARTESIAN_POINT('',(2.55,1.,0.7));
#21525=CARTESIAN_POINT('Origin',(2.7,1.,0.7));
#21526=CARTESIAN_POINT('Origin',(2.7,1.,0.7));
#21527=CARTESIAN_POINT('',(2.45,1.,0.6));
#21528=CARTESIAN_POINT('Origin',(2.7,1.,0.6));
#21529=CARTESIAN_POINT('',(2.45,1.,0.7));
#21530=CARTESIAN_POINT('Origin',(2.7,1.,0.6));
#21531=CARTESIAN_POINT('Origin',(8.1,-1.,0.7));
#21532=CARTESIAN_POINT('',(7.85,-1.,0.7));
#21533=CARTESIAN_POINT('Origin',(8.1,-1.,0.7));
#21534=CARTESIAN_POINT('',(7.95,-1.,0.7));
#21535=CARTESIAN_POINT('Origin',(8.1,-1.,0.7));
#21536=CARTESIAN_POINT('Origin',(8.1,-1.,0.7));
#21537=CARTESIAN_POINT('',(7.85,-1.,0.6));
#21538=CARTESIAN_POINT('Origin',(8.1,-1.,0.6));
#21539=CARTESIAN_POINT('',(7.85,-1.,0.7));
#21540=CARTESIAN_POINT('Origin',(8.1,-1.,0.6));
#21541=CARTESIAN_POINT('Origin',(8.1,1.,0.9));
#21542=CARTESIAN_POINT('',(7.95,1.,0.9));
#21543=CARTESIAN_POINT('',(7.95,1.,0.9));
#21544=CARTESIAN_POINT('Origin',(8.1,1.,0.9));
#21545=CARTESIAN_POINT('Origin',(2.7,-1.,0.9));
#21546=CARTESIAN_POINT('',(2.55,-1.,0.9));
#21547=CARTESIAN_POINT('',(2.55,-1.,0.9));
#21548=CARTESIAN_POINT('Origin',(2.7,-1.,0.9));
#21549=CARTESIAN_POINT('Origin',(2.7,1.,0.9));
#21550=CARTESIAN_POINT('',(2.55,1.,0.9));
#21551=CARTESIAN_POINT('',(2.55,1.,0.9));
#21552=CARTESIAN_POINT('Origin',(2.7,1.,0.9));
#21553=CARTESIAN_POINT('Origin',(8.1,-1.,0.9));
#21554=CARTESIAN_POINT('',(7.95,-1.,0.9));
#21555=CARTESIAN_POINT('',(7.95,-1.,0.9));
#21556=CARTESIAN_POINT('Origin',(8.1,-1.,0.9));
#21557=CARTESIAN_POINT('Ctrl Pts',(10.3006295894369,0.974894988741159,1.1));
#21558=CARTESIAN_POINT('Ctrl Pts',(10.315705472156,0.974011521809381,1.1));
#21559=CARTESIAN_POINT('Ctrl Pts',(10.3502474882039,0.960160784532573,1.1));
#21560=CARTESIAN_POINT('Ctrl Pts',(10.3664342774515,0.92524659453289,1.1));
#21561=CARTESIAN_POINT('Ctrl Pts',(10.3664342774515,0.905110932257975,1.1));
#21562=CARTESIAN_POINT('Ctrl Pts',(10.3019806204244,0.997949597787003,1.1));
#21563=CARTESIAN_POINT('Ctrl Pts',(10.3220349090938,0.996609784625678,1.09999398337427));
#21564=CARTESIAN_POINT('Ctrl Pts',(10.3677183242066,0.978025516808524,1.09998506712737));
#21565=CARTESIAN_POINT('Ctrl Pts',(10.3893396302527,0.931918448901421,1.09999143472557));
#21566=CARTESIAN_POINT('Ctrl Pts',(10.3895723566779,0.905110932257975,1.1));
#21567=CARTESIAN_POINT('Ctrl Pts',(10.3043223099121,1.03790925537118,1.08136572286424));
#21568=CARTESIAN_POINT('Ctrl Pts',(10.3329503749445,1.0358015962555,1.08164234815929));
#21569=CARTESIAN_POINT('Ctrl Pts',(10.3979372989902,1.00899285190124,1.08203919297574));
#21570=CARTESIAN_POINT('Ctrl Pts',(10.4290660105163,0.943405843911333,1.08168333012239));
#21571=CARTESIAN_POINT('Ctrl Pts',(10.4296737498558,0.905110932257975,1.08129070628762));
#21572=CARTESIAN_POINT('Ctrl Pts',(10.3052465815697,1.05368144854439,1.04171131144128));
#21573=CARTESIAN_POINT('Ctrl Pts',(10.3373036016374,1.05157771141627,1.04242733672965));
#21574=CARTESIAN_POINT('Ctrl Pts',(10.4104769365187,1.02185126978705,1.04346621563788));
#21575=CARTESIAN_POINT('Ctrl Pts',(10.445100550936,0.94795146444073,1.04253150017828));
#21576=CARTESIAN_POINT('Ctrl Pts',(10.4454164251054,0.905110932257975,1.0415166534692));
#21577=CARTESIAN_POINT('Ctrl Pts',(10.3053025283406,1.05463614976313,1.02441711227736));
#21578=CARTESIAN_POINT('Ctrl Pts',(10.3375636805833,1.05269876817044,1.02526261130878));
#21579=CARTESIAN_POINT('Ctrl Pts',(10.411517621087,1.0229540574362,1.02649649899074));
#21580=CARTESIAN_POINT('Ctrl Pts',(10.4462618831994,0.948196125723061,1.02538435201347));
#21581=CARTESIAN_POINT('Ctrl Pts',(10.4463246402318,0.905110932257975,1.02418687649944));
#21582=CARTESIAN_POINT('',(10.3664342774515,0.905110932257975,1.1));
#21583=CARTESIAN_POINT('',(10.4463246402318,0.905110932257975,1.02418687649943));
#21584=CARTESIAN_POINT('Origin',(10.3664342774515,0.905110932257975,1.02));
#21585=CARTESIAN_POINT('',(10.3053025283406,1.05463614976313,1.02441711227738));
#21586=CARTESIAN_POINT('Ctrl Pts',(10.4463246402318,0.905110932257975,1.02418687649944));
#21587=CARTESIAN_POINT('Ctrl Pts',(10.4462618831994,0.948196125723061,1.02538435201347));
#21588=CARTESIAN_POINT('Ctrl Pts',(10.411517621087,1.0229540574362,1.02649649899074));
#21589=CARTESIAN_POINT('Ctrl Pts',(10.3375636805833,1.05269876817044,1.02526261130878));
#21590=CARTESIAN_POINT('Ctrl Pts',(10.3053025283406,1.05463614976313,1.02441711227736));
#21591=CARTESIAN_POINT('',(10.3006295894369,0.974894988741159,1.1));
#21592=CARTESIAN_POINT('Origin',(10.3006295894369,0.974894988741159,1.02));
#21593=CARTESIAN_POINT('Ctrl Pts',(10.3006295894369,0.974894988741159,1.1));
#21594=CARTESIAN_POINT('Ctrl Pts',(10.315705472156,0.974011521809381,1.1));
#21595=CARTESIAN_POINT('Ctrl Pts',(10.3502474882039,0.960160784532573,1.1));
#21596=CARTESIAN_POINT('Ctrl Pts',(10.3664342774515,0.92524659453289,1.1));
#21597=CARTESIAN_POINT('Ctrl Pts',(10.3664342774515,0.905110932257975,1.1));
#21598=CARTESIAN_POINT('Origin',(10.3664342774515,0.526416499322631,1.02));
#21599=CARTESIAN_POINT('',(10.3664342774515,-0.905110932257974,1.1));
#21600=CARTESIAN_POINT('',(10.4463246402318,-0.905110932257974,1.02418687649944));
#21601=CARTESIAN_POINT('Origin',(10.3664342774515,-0.905110932257974,1.02));
#21602=CARTESIAN_POINT('',(10.4463246402318,0.526416499322631,1.02418687649944));
#21603=CARTESIAN_POINT('',(10.3664342774515,0.526416499322631,1.1));
#21604=CARTESIAN_POINT('Ctrl Pts',(10.3664342774515,-0.905110932257974,
1.1));
#21605=CARTESIAN_POINT('Ctrl Pts',(10.3664342774515,-0.920212678972614,
1.1));
#21606=CARTESIAN_POINT('Ctrl Pts',(10.3546350195413,-0.955507038097987,
1.1));
#21607=CARTESIAN_POINT('Ctrl Pts',(10.3207307664069,-0.973717032831462,
1.1));
#21608=CARTESIAN_POINT('Ctrl Pts',(10.3006295894369,-0.974894988741159,
1.1));
#21609=CARTESIAN_POINT('Ctrl Pts',(10.3895723566779,-0.905110932257974,
1.1));
#21610=CARTESIAN_POINT('Ctrl Pts',(10.3893978118589,-0.925216569751813,
1.09999357604418));
#21611=CARTESIAN_POINT('Ctrl Pts',(10.3734893817427,-0.971910228734235,
1.09998467394719));
#21612=CARTESIAN_POINT('Ctrl Pts',(10.3287196719985,-0.996163180237569,
1.09999197783236));
#21613=CARTESIAN_POINT('Ctrl Pts',(10.3019806204244,-0.997949597787003,
1.1));
#21614=CARTESIAN_POINT('Ctrl Pts',(10.4296737498558,-0.905110932257974,
1.0812907062876));
#21615=CARTESIAN_POINT('Ctrl Pts',(10.4292179453509,-0.933832116014069,
1.08158517416384));
#21616=CARTESIAN_POINT('Ctrl Pts',(10.4061705706524,-1.00027633256302,1.08203447943735));
#21617=CARTESIAN_POINT('Ctrl Pts',(10.3424930633099,-1.03509904321534,1.08173455659116));
#21618=CARTESIAN_POINT('Ctrl Pts',(10.3043223099121,-1.03790925537115,1.08136572286421));
#21619=CARTESIAN_POINT('Ctrl Pts',(10.4454164251054,-0.905110932257974,
1.0415166534692));
#21620=CARTESIAN_POINT('Ctrl Pts',(10.4451795194782,-0.937241331413026,
1.04227778850144));
#21621=CARTESIAN_POINT('Ctrl Pts',(10.4197512278104,-1.01202259423409,1.0434534732467));
#21622=CARTESIAN_POINT('Ctrl Pts',(10.3479892750172,-1.05087646570533,1.0426660118263));
#21623=CARTESIAN_POINT('Ctrl Pts',(10.3052465815697,-1.05368144854438,1.04171131144128));
#21624=CARTESIAN_POINT('Ctrl Pts',(10.4463246402318,-0.905110932257974,
1.02418687649944));
#21625=CARTESIAN_POINT('Ctrl Pts',(10.4462775724575,-0.937424827374877,
1.02508498313546));
#21626=CARTESIAN_POINT('Ctrl Pts',(10.4209202812412,-1.01298254961426,1.02648109501254));
#21627=CARTESIAN_POINT('Ctrl Pts',(10.3483173980216,-1.05205297430477,1.02554444431988));
#21628=CARTESIAN_POINT('Ctrl Pts',(10.3053025283406,-1.05463614976313,1.02441711227736));
#21629=CARTESIAN_POINT('',(10.3006295894369,-0.974894988741159,1.1));
#21630=CARTESIAN_POINT('',(10.3053025283406,-1.05463614976313,1.02441711227736));
#21631=CARTESIAN_POINT('Origin',(10.3006295894369,-0.974894988741159,1.02));
#21632=CARTESIAN_POINT('Ctrl Pts',(10.3053025283406,-1.05463614976313,1.02441711227736));
#21633=CARTESIAN_POINT('Ctrl Pts',(10.3483173980216,-1.05205297430477,1.02554444431988));
#21634=CARTESIAN_POINT('Ctrl Pts',(10.4209202812412,-1.01298254961426,1.02648109501254));
#21635=CARTESIAN_POINT('Ctrl Pts',(10.4462775724575,-0.937424827374877,
1.02508498313546));
#21636=CARTESIAN_POINT('Ctrl Pts',(10.4463246402318,-0.905110932257974,
1.02418687649944));
#21637=CARTESIAN_POINT('Ctrl Pts',(10.3664342774515,-0.905110932257974,
1.1));
#21638=CARTESIAN_POINT('Ctrl Pts',(10.3664342774515,-0.920212678972614,
1.1));
#21639=CARTESIAN_POINT('Ctrl Pts',(10.3546350195413,-0.955507038097987,
1.1));
#21640=CARTESIAN_POINT('Ctrl Pts',(10.3207307664069,-0.973717032831462,
1.1));
#21641=CARTESIAN_POINT('Ctrl Pts',(10.3006295894369,-0.974894988741159,
1.1));
#21642=CARTESIAN_POINT('Ctrl Pts',(10.3006295894369,-0.974894988741159,
1.1));
#21643=CARTESIAN_POINT('Ctrl Pts',(8.90133038997308,-1.05689579714676,1.1));
#21644=CARTESIAN_POINT('Ctrl Pts',(5.63386529032775,-1.20659234980357,1.1));
#21645=CARTESIAN_POINT('Ctrl Pts',(2.35953432096223,-1.1387902266302,1.1));
#21646=CARTESIAN_POINT('Ctrl Pts',(0.497468741075922,-0.978719373910683,
1.1));
#21647=CARTESIAN_POINT('Ctrl Pts',(10.3019806204244,-0.997949597787003,
1.1));
#21648=CARTESIAN_POINT('Ctrl Pts',(8.90248440956766,-1.07998148241326,1.10000071389857));
#21649=CARTESIAN_POINT('Ctrl Pts',(5.63428345559727,-1.22975661509925,1.09999860206726));
#21650=CARTESIAN_POINT('Ctrl Pts',(2.35854977485598,-1.16192218645588,1.10000206853834));
#21651=CARTESIAN_POINT('Ctrl Pts',(0.495492436783665,-1.00170924455528,
1.1));
#21652=CARTESIAN_POINT('Ctrl Pts',(10.3043223112023,-1.03790927738781,1.08136574244164));
#21653=CARTESIAN_POINT('Ctrl Pts',(8.90448672538924,-1.11999254202045,1.08133291965814));
#21654=CARTESIAN_POINT('Ctrl Pts',(5.63501252140964,-1.26990499402305,1.08126385742935));
#21655=CARTESIAN_POINT('Ctrl Pts',(2.35683262246169,-1.20200947624765,1.08130376582018));
#21656=CARTESIAN_POINT('Ctrl Pts',(0.492066872450609,-1.0415580073244,1.08139899772624));
#21657=CARTESIAN_POINT('Ctrl Pts',(10.3052465815697,-1.05368144854439,1.04171131144128));
#21658=CARTESIAN_POINT('Ctrl Pts',(8.90527383415966,-1.13574844311122,1.04162635195479));
#21659=CARTESIAN_POINT('Ctrl Pts',(5.63529344743191,-1.28563363803111,1.04144655753461));
#21660=CARTESIAN_POINT('Ctrl Pts',(2.35616768559357,-1.21776439538312,1.04155103737704));
#21661=CARTESIAN_POINT('Ctrl Pts',(0.490711556403977,-1.05732407164794,
1.04179769276967));
#21662=CARTESIAN_POINT('Ctrl Pts',(10.3053025283406,-1.05463614976313,1.02441711227736));
#21663=CARTESIAN_POINT('Ctrl Pts',(8.90532084970199,-1.13668250951809,1.02431679017323));
#21664=CARTESIAN_POINT('Ctrl Pts',(5.63530902077156,-1.28652517622799,1.02410366945797));
#21665=CARTESIAN_POINT('Ctrl Pts',(2.35612886002319,-1.2186808487933,1.02422798328229));
#21666=CARTESIAN_POINT('Ctrl Pts',(0.490627822843887,-1.05829812393464,
1.02451933428366));
#21667=CARTESIAN_POINT('',(0.497468741075922,-0.978719373910683,1.1));
#21668=CARTESIAN_POINT('',(0.490627822843887,-1.05829812393464,1.02451933428366));
#21669=CARTESIAN_POINT('Origin',(0.497468741075922,-0.978719373910683,1.02));
#21670=CARTESIAN_POINT('Ctrl Pts',(0.490627822843887,-1.05829812393464,
1.02451933428366));
#21671=CARTESIAN_POINT('Ctrl Pts',(2.35612886002319,-1.2186808487933,1.02422798328229));
#21672=CARTESIAN_POINT('Ctrl Pts',(5.63530902077156,-1.28652517622799,1.02410366945797));
#21673=CARTESIAN_POINT('Ctrl Pts',(8.90532084970199,-1.13668250951809,1.02431679017323));
#21674=CARTESIAN_POINT('Ctrl Pts',(10.3053025283406,-1.05463614976313,1.02441711227736));
#21675=CARTESIAN_POINT('Ctrl Pts',(10.3006295894369,-0.974894988741159,
1.1));
#21676=CARTESIAN_POINT('Ctrl Pts',(8.90133038997308,-1.05689579714676,1.1));
#21677=CARTESIAN_POINT('Ctrl Pts',(5.63386529032775,-1.20659234980357,1.1));
#21678=CARTESIAN_POINT('Ctrl Pts',(2.35953432096223,-1.1387902266302,1.1));
#21679=CARTESIAN_POINT('Ctrl Pts',(0.497468741075922,-0.978719373910683,
1.1));
#21680=CARTESIAN_POINT('Ctrl Pts',(0.497468741075921,-0.978719373910683,
1.1));
#21681=CARTESIAN_POINT('Ctrl Pts',(0.482693827936028,-0.977449261315989,
1.1));
#21682=CARTESIAN_POINT('Ctrl Pts',(0.449140492346353,-0.963153189418853,
1.1));
#21683=CARTESIAN_POINT('Ctrl Pts',(0.433565722548535,-0.928845297374623,
1.1));
#21684=CARTESIAN_POINT('Ctrl Pts',(0.433565722548535,-0.909072757750428,
1.1));
#21685=CARTESIAN_POINT('Ctrl Pts',(0.495492436783665,-1.00170924455528,
1.1));
#21686=CARTESIAN_POINT('Ctrl Pts',(0.475845599502289,-0.99986336234735,
1.09999428725696));
#21687=CARTESIAN_POINT('Ctrl Pts',(0.431470670910625,-0.980707626108276,
1.09998595101222));
#21688=CARTESIAN_POINT('Ctrl Pts',(0.410656014536328,-0.935396857641307,
1.09999159501496));
#21689=CARTESIAN_POINT('Ctrl Pts',(0.410427643322096,-0.909072757750428,
1.1));
#21690=CARTESIAN_POINT('Ctrl Pts',(0.492065445269591,-1.04157460937658,
1.08141381101793));
#21691=CARTESIAN_POINT('Ctrl Pts',(0.464027324938814,-1.03875422423143,
1.08167681576789));
#21692=CARTESIAN_POINT('Ctrl Pts',(0.400896096452139,-1.01114975683443,
1.0820463630617));
#21693=CARTESIAN_POINT('Ctrl Pts',(0.370905720538455,-0.946677133941945,
1.08169093175476));
#21694=CARTESIAN_POINT('Ctrl Pts',(0.370309354350991,-0.909072757750428,
1.08130565542949));
#21695=CARTESIAN_POINT('Ctrl Pts',(0.490711556403977,-1.05732407164794,
1.04179769276967));
#21696=CARTESIAN_POINT('Ctrl Pts',(0.459302109313527,-1.05440855600651,
1.04247888820671));
#21697=CARTESIAN_POINT('Ctrl Pts',(0.388222412631638,-1.02376232464153,
1.04344633806995));
#21698=CARTESIAN_POINT('Ctrl Pts',(0.354893537837358,-0.951140796546497,
1.04251250847383));
#21699=CARTESIAN_POINT('Ctrl Pts',(0.354583574894625,-0.909072757750428,
1.0415166534692));
#21700=CARTESIAN_POINT('Ctrl Pts',(0.490627822843887,-1.05829812393464,
1.02451933428366));
#21701=CARTESIAN_POINT('Ctrl Pts',(0.459009463695281,-1.05553438344805,
1.02532396689517));
#21702=CARTESIAN_POINT('Ctrl Pts',(0.387169680965019,-1.0248398620393,1.02647307310763));
#21703=CARTESIAN_POINT('Ctrl Pts',(0.353736942373964,-0.951381046565094,
1.02536194261819));
#21704=CARTESIAN_POINT('Ctrl Pts',(0.35367535976817,-0.909072757750428,
1.02418687649944));
#21705=CARTESIAN_POINT('',(0.433565722548535,-0.909072757750428,1.1));
#21706=CARTESIAN_POINT('',(0.35367535976817,-0.909072757750428,1.02418687649944));
#21707=CARTESIAN_POINT('Origin',(0.433565722548536,-0.909072757750428,1.02));
#21708=CARTESIAN_POINT('Ctrl Pts',(0.35367535976817,-0.909072757750428,
1.02418687649944));
#21709=CARTESIAN_POINT('Ctrl Pts',(0.353736942373964,-0.951381046565094,
1.02536194261819));
#21710=CARTESIAN_POINT('Ctrl Pts',(0.387169680965019,-1.0248398620393,1.02647307310763));
#21711=CARTESIAN_POINT('Ctrl Pts',(0.459009463695281,-1.05553438344805,
1.02532396689517));
#21712=CARTESIAN_POINT('Ctrl Pts',(0.490627822843887,-1.05829812393464,
1.02451933428366));
#21713=CARTESIAN_POINT('Ctrl Pts',(0.497468741075921,-0.978719373910683,
1.1));
#21714=CARTESIAN_POINT('Ctrl Pts',(0.482693827936028,-0.977449261315989,
1.1));
#21715=CARTESIAN_POINT('Ctrl Pts',(0.449140492346353,-0.963153189418853,
1.1));
#21716=CARTESIAN_POINT('Ctrl Pts',(0.433565722548535,-0.928845297374623,
1.1));
#21717=CARTESIAN_POINT('Ctrl Pts',(0.433565722548535,-0.909072757750428,
1.1));
#21718=CARTESIAN_POINT('Origin',(0.433565722548535,-0.526416499322631,1.02));
#21719=CARTESIAN_POINT('',(0.433565722548535,0.909072757750428,1.1));
#21720=CARTESIAN_POINT('',(0.35367535976817,0.909072757750428,1.02418687649944));
#21721=CARTESIAN_POINT('Origin',(0.433565722548535,0.909072757750428,1.02));
#21722=CARTESIAN_POINT('',(0.35367535976817,-0.526416499322631,1.02418687649944));
#21723=CARTESIAN_POINT('',(0.433565722548535,-0.526416499322631,1.1));
#21724=CARTESIAN_POINT('Ctrl Pts',(0.433565722548535,0.909072757750428,
1.1));
#21725=CARTESIAN_POINT('Ctrl Pts',(0.433565722548535,0.923902162481473,
1.1));
#21726=CARTESIAN_POINT('Ctrl Pts',(0.444925688709976,0.95855828847753,1.1));
#21727=CARTESIAN_POINT('Ctrl Pts',(0.477768856872263,0.977025890449618,
1.1));
#21728=CARTESIAN_POINT('Ctrl Pts',(0.497468741075922,0.978719373910683,
1.1));
#21729=CARTESIAN_POINT('Ctrl Pts',(0.410427643322096,0.909072757750428,
1.1));
#21730=CARTESIAN_POINT('Ctrl Pts',(0.410598921732919,0.928815832685761,
1.09999369626122));
#21731=CARTESIAN_POINT('Ctrl Pts',(0.425924740546694,0.974670094016788,
1.09998538828789));
#21732=CARTESIAN_POINT('Ctrl Pts',(0.469296653719046,0.9992480682759,1.09999238300928));
#21733=CARTESIAN_POINT('Ctrl Pts',(0.495492436783666,1.00170924455528,1.1));
#21734=CARTESIAN_POINT('Ctrl Pts',(0.370309354350991,0.909072757750428,
1.08130565542949));
#21735=CARTESIAN_POINT('Ctrl Pts',(0.370756628991978,0.937276039918598,
1.0815946126737));
#21736=CARTESIAN_POINT('Ctrl Pts',(0.392976709797646,1.00253976529927,1.08203966084696));
#21737=CARTESIAN_POINT('Ctrl Pts',(0.45468128479604,1.03781409584644,1.08176448401818));
#21738=CARTESIAN_POINT('Ctrl Pts',(0.492065445269591,1.04157460937658,1.08141381101793));
#21739=CARTESIAN_POINT('Ctrl Pts',(0.354583574894625,0.909072757750428,
1.0415166534692));
#21740=CARTESIAN_POINT('Ctrl Pts',(0.354816047101877,0.940623786874923,
1.04226354472332));
#21741=CARTESIAN_POINT('Ctrl Pts',(0.379310481833935,1.01405872099115,1.04342813304911));
#21742=CARTESIAN_POINT('Ctrl Pts',(0.448832293580285,1.05343671745598,1.04270595335318));
#21743=CARTESIAN_POINT('Ctrl Pts',(0.490711556403977,1.05732407164794,1.04179769276967));
#21744=CARTESIAN_POINT('Ctrl Pts',(0.35367535976817,0.909072757750428,1.02418687649944));
#21745=CARTESIAN_POINT('Ctrl Pts',(0.353721546722556,0.940803974389028,
1.02506817608927));
#21746=CARTESIAN_POINT('Ctrl Pts',(0.378136805744942,1.01499479618886,1.02645106984513));
#21747=CARTESIAN_POINT('Ctrl Pts',(0.448470010609076,1.05461313661598,1.0255921777666));
#21748=CARTESIAN_POINT('Ctrl Pts',(0.490627822843887,1.05829812393464,1.02451933428366));
#21749=CARTESIAN_POINT('',(0.497468741075921,0.978719373910683,1.1));
#21750=CARTESIAN_POINT('',(0.490627822843887,1.05829812393464,1.02451933428366));
#21751=CARTESIAN_POINT('Origin',(0.497468741075921,0.978719373910683,1.02));
#21752=CARTESIAN_POINT('Ctrl Pts',(0.490627822843887,1.05829812393464,1.02451933428366));
#21753=CARTESIAN_POINT('Ctrl Pts',(0.448470010609076,1.05461313661598,1.0255921777666));
#21754=CARTESIAN_POINT('Ctrl Pts',(0.378136805744942,1.01499479618886,1.02645106984513));
#21755=CARTESIAN_POINT('Ctrl Pts',(0.353721546722556,0.940803974389028,
1.02506817608927));
#21756=CARTESIAN_POINT('Ctrl Pts',(0.35367535976817,0.909072757750428,1.02418687649944));
#21757=CARTESIAN_POINT('Ctrl Pts',(0.433565722548535,0.909072757750428,
1.1));
#21758=CARTESIAN_POINT('Ctrl Pts',(0.433565722548535,0.923902162481473,
1.1));
#21759=CARTESIAN_POINT('Ctrl Pts',(0.444925688709976,0.95855828847753,1.1));
#21760=CARTESIAN_POINT('Ctrl Pts',(0.477768856872263,0.977025890449618,
1.1));
#21761=CARTESIAN_POINT('Ctrl Pts',(0.497468741075922,0.978719373910683,
1.1));
#21762=CARTESIAN_POINT('Ctrl Pts',(0.497468741075922,0.978719373910683,
1.1));
#21763=CARTESIAN_POINT('Ctrl Pts',(1.89401780684616,1.09877250320817,1.1));
#21764=CARTESIAN_POINT('Ctrl Pts',(5.1654052076905,1.21987569230965,1.1));
#21765=CARTESIAN_POINT('Ctrl Pts',(8.43489748265729,1.08422939062092,1.1));
#21766=CARTESIAN_POINT('Ctrl Pts',(10.3006295894369,0.974894988741159,1.1));
#21767=CARTESIAN_POINT('Ctrl Pts',(0.495492436783665,1.00170924455528,1.1));
#21768=CARTESIAN_POINT('Ctrl Pts',(1.89278532112995,1.12186894072949,1.10000155140362));
#21769=CARTESIAN_POINT('Ctrl Pts',(5.16566149651331,1.24305592512388,1.09999870932828));
#21770=CARTESIAN_POINT('Ctrl Pts',(8.43598583180997,1.1073254346241,1.10000095186468));
#21771=CARTESIAN_POINT('Ctrl Pts',(10.3019806204244,0.997949597787003,1.1));
#21772=CARTESIAN_POINT('Ctrl Pts',(0.492066872450609,1.0415580073244,1.08139899772624));
#21773=CARTESIAN_POINT('Ctrl Pts',(1.89064106564166,1.16189659875033,1.08132757380279));
#21774=CARTESIAN_POINT('Ctrl Pts',(5.16610832342906,1.28323142649893,1.0812556832418));
#21775=CARTESIAN_POINT('Ctrl Pts',(8.43787502268472,1.14735362089424,1.08132197873404));
#21776=CARTESIAN_POINT('Ctrl Pts',(10.3043223112023,1.03790927738781,1.08136574244164));
#21777=CARTESIAN_POINT('Ctrl Pts',(0.490711556403977,1.05732407164794,1.04179769276967));
#21778=CARTESIAN_POINT('Ctrl Pts',(1.88980353393473,1.17765430418353,1.04161270124098));
#21779=CARTESIAN_POINT('Ctrl Pts',(5.16628155123749,1.29896165650174,1.04142536433641));
#21780=CARTESIAN_POINT('Ctrl Pts',(8.43861641093843,1.16310409863161,1.04159803213562));
#21781=CARTESIAN_POINT('Ctrl Pts',(10.3052465815697,1.05368144854439,1.04171131144128));
#21782=CARTESIAN_POINT('Ctrl Pts',(0.490627822843887,1.05829812393464,1.02451933428366));
#21783=CARTESIAN_POINT('Ctrl Pts',(1.88975348136405,1.17858515731652,1.02430082105127));
#21784=CARTESIAN_POINT('Ctrl Pts',(5.16629169073646,1.29984841142479,1.02407861909595));
#21785=CARTESIAN_POINT('Ctrl Pts',(8.43866044940558,1.1640312867702,1.02428334948326));
#21786=CARTESIAN_POINT('Ctrl Pts',(10.3053025283406,1.05463614976313,1.02441711227736));
#21787=CARTESIAN_POINT('Ctrl Pts',(10.3053025283406,1.05463614976313,1.02441711227736));
#21788=CARTESIAN_POINT('Ctrl Pts',(8.43866044940558,1.1640312867702,1.02428334948326));
#21789=CARTESIAN_POINT('Ctrl Pts',(5.16629169073646,1.29984841142479,1.02407861909595));
#21790=CARTESIAN_POINT('Ctrl Pts',(1.88975348136405,1.17858515731652,1.02430082105127));
#21791=CARTESIAN_POINT('Ctrl Pts',(0.490627822843887,1.05829812393464,1.02451933428366));
#21792=CARTESIAN_POINT('Ctrl Pts',(0.497468741075922,0.978719373910683,
1.1));
#21793=CARTESIAN_POINT('Ctrl Pts',(1.89401780684616,1.09877250320817,1.1));
#21794=CARTESIAN_POINT('Ctrl Pts',(5.1654052076905,1.21987569230965,1.1));
#21795=CARTESIAN_POINT('Ctrl Pts',(8.43489748265729,1.08422939062092,1.1));
#21796=CARTESIAN_POINT('Ctrl Pts',(10.3006295894369,0.974894988741159,1.1));
#21797=CARTESIAN_POINT('Origin',(0.347167001354737,-1.05283299864526,0.9));
#21798=CARTESIAN_POINT('',(0.347167001354737,0.915565952400859,0.9));
#21799=CARTESIAN_POINT('Ctrl Pts',(0.347167001354737,0.915565952400859,
0.9));
#21800=CARTESIAN_POINT('Ctrl Pts',(0.349336454142569,0.913401548092598,
0.941395625182189));
#21801=CARTESIAN_POINT('Ctrl Pts',(0.351505906947026,0.911237149868421,
0.982791250681617));
#21802=CARTESIAN_POINT('Ctrl Pts',(0.35367535976817,0.909072757750428,1.02418687649944));
#21803=CARTESIAN_POINT('',(0.347167001354737,-0.915565952400859,0.9));
#21804=CARTESIAN_POINT('',(0.347167001354737,-1.05283299864526,0.9));
#21805=CARTESIAN_POINT('Ctrl Pts',(0.35367535976817,-0.909072757750428,
1.02418687649944));
#21806=CARTESIAN_POINT('Ctrl Pts',(0.351505906947026,-0.911237149868421,
0.982791250681617));
#21807=CARTESIAN_POINT('Ctrl Pts',(0.349336454142569,-0.913401548092598,
0.941395625182188));
#21808=CARTESIAN_POINT('Ctrl Pts',(0.347167001354737,-0.915565952400859,
0.9));
#21809=CARTESIAN_POINT('Ctrl Pts',(0.346993933238254,0.915738617787778,
0.896697663613103));
#21810=CARTESIAN_POINT('Ctrl Pts',(0.349221075397351,0.913516658022686,
0.939194067573829));
#21811=CARTESIAN_POINT('Ctrl Pts',(0.351448217573968,0.911294704668933,
0.981690471868858));
#21812=CARTESIAN_POINT('Ctrl Pts',(0.35367535976817,0.909072757750428,1.02418687649944));
#21813=CARTESIAN_POINT('Ctrl Pts',(0.3471095194732,0.958036394339727,0.898903180361322));
#21814=CARTESIAN_POINT('Ctrl Pts',(0.349336694827029,0.955813381999015,
0.941399523267081));
#21815=CARTESIAN_POINT('Ctrl Pts',(0.351563761373338,0.953590428181058,
0.983895874971515));
#21816=CARTESIAN_POINT('Ctrl Pts',(0.353790936839104,0.951367426011707,
1.0263922183879));
#21817=CARTESIAN_POINT('Ctrl Pts',(0.38058410360499,1.03143776743275,0.900986703480571));
#21818=CARTESIAN_POINT('Ctrl Pts',(0.382809509257377,1.02921304595835,0.943483042387942));
#21819=CARTESIAN_POINT('Ctrl Pts',(0.38503494445329,1.0269883029847,0.985979378580876));
#21820=CARTESIAN_POINT('Ctrl Pts',(0.38726034587086,1.02476358729949,1.02847571797107));
#21821=CARTESIAN_POINT('Ctrl Pts',(0.452370958194108,1.06215086202928,0.898830373501354));
#21822=CARTESIAN_POINT('Ctrl Pts',(0.454593549384999,1.0599273359084,0.941326919294252));
#21823=CARTESIAN_POINT('Ctrl Pts',(0.456816159498039,1.05770384366995,0.983823465869046));
#21824=CARTESIAN_POINT('Ctrl Pts',(0.459038739297573,1.0554803259981,1.02632001264655));
#21825=CARTESIAN_POINT('Ctrl Pts',(0.48397786901498,1.06495020962439,0.897320291708494));
#21826=CARTESIAN_POINT('Ctrl Pts',(0.486199596570706,1.06272777115298,0.939816939358577));
#21827=CARTESIAN_POINT('Ctrl Pts',(0.488421317286976,1.06050533819043,0.982313587627295));
#21828=CARTESIAN_POINT('Ctrl Pts',(0.49064303113777,1.05828291075608,1.02481023651688));
#21829=CARTESIAN_POINT('',(0.484117964332956,1.06481006947648,0.9));
#21830=CARTESIAN_POINT('Ctrl Pts',(0.490627822843887,1.05829812393464,1.02451933428366));
#21831=CARTESIAN_POINT('Ctrl Pts',(0.488457876548035,1.06046876718106,0.983012888930869));
#21832=CARTESIAN_POINT('Ctrl Pts',(0.486287923702977,1.06263941570101,0.941506444170341));
#21833=CARTESIAN_POINT('Ctrl Pts',(0.484117964332956,1.06481006947648,0.9));
#21834=CARTESIAN_POINT('Ctrl Pts',(0.484117964332956,1.06481006947648,0.9));
#21835=CARTESIAN_POINT('Ctrl Pts',(0.473400395954556,1.06388989254567,0.899999999998067));
#21836=CARTESIAN_POINT('Ctrl Pts',(0.462835544435657,1.06178983909504,0.899998456484708));
#21837=CARTESIAN_POINT('Ctrl Pts',(0.452598733053303,1.05860868771556,0.899998088469989));
#21838=CARTESIAN_POINT('Ctrl Pts',(0.444242646677269,1.05601198306707,0.899997788067582));
#21839=CARTESIAN_POINT('Ctrl Pts',(0.436104524303727,1.05269365102958,0.899998236040192));
#21840=CARTESIAN_POINT('Ctrl Pts',(0.428287607266336,1.04868302953039,0.899999222960128));
#21841=CARTESIAN_POINT('Ctrl Pts',(0.418720381516705,1.0437743780639,0.900000430864189));
#21842=CARTESIAN_POINT('Ctrl Pts',(0.409734998843702,1.03788190267505,0.900002558923036));
#21843=CARTESIAN_POINT('Ctrl Pts',(0.401509364000825,1.03108161209803,0.900001877425249));
#21844=CARTESIAN_POINT('Ctrl Pts',(0.400282968007853,1.0300677269361,0.900001775817754));
#21845=CARTESIAN_POINT('Ctrl Pts',(0.399073506836177,1.02903357975146,0.900001605039306));
#21846=CARTESIAN_POINT('Ctrl Pts',(0.397881626738084,1.02797933950107,0.900001345423406));
#21847=CARTESIAN_POINT('Ctrl Pts',(0.39256805719391,1.02327938780652,0.900000188019117));
#21848=CARTESIAN_POINT('Ctrl Pts',(0.387603264903844,1.01818054769329,0.899997323013939));
#21849=CARTESIAN_POINT('Ctrl Pts',(0.383010638913681,1.01272978836618,0.899994456107983));
#21850=CARTESIAN_POINT('Ctrl Pts',(0.37606924632558,1.00449139480359,0.899990123005355));
#21851=CARTESIAN_POINT('Ctrl Pts',(0.370046554889952,0.995534526609835,
0.899986018340436));
#21852=CARTESIAN_POINT('Ctrl Pts',(0.3650033874046,0.986038739193365,0.899984773108821));
#21853=CARTESIAN_POINT('Ctrl Pts',(0.361794276996282,0.979996300523246,
0.899983980732651));
#21854=CARTESIAN_POINT('Ctrl Pts',(0.358982518390177,0.973734765189587,
0.899984261914926));
#21855=CARTESIAN_POINT('Ctrl Pts',(0.356593362150852,0.967295151176304,
0.899985518247832));
#21856=CARTESIAN_POINT('Ctrl Pts',(0.352862932284158,0.957240334312622,
0.899987479886722));
#21857=CARTESIAN_POINT('Ctrl Pts',(0.350196128254646,0.946848238515865,
0.899991935314924));
#21858=CARTESIAN_POINT('Ctrl Pts',(0.348668140386249,0.936282377262574,
0.899995621109591));
#21859=CARTESIAN_POINT('Ctrl Pts',(0.347678076093379,0.929436195976283,
0.89999800933123));
#21860=CARTESIAN_POINT('Ctrl Pts',(0.347167001781036,0.922516504287413,
0.899999999966543));
#21861=CARTESIAN_POINT('Ctrl Pts',(0.347167001354737,0.915565952400859,
0.9));
#21862=CARTESIAN_POINT('Ctrl Pts',(0.484117964332956,1.06481006947648,0.9));
#21863=CARTESIAN_POINT('Ctrl Pts',(0.486234267105875,1.06263480888061,0.94150644476122));
#21864=CARTESIAN_POINT('Ctrl Pts',(0.488350569878795,1.06045954828474,0.98301288952244));
#21865=CARTESIAN_POINT('Ctrl Pts',(0.490466872651714,1.05828428768887,1.02451933428366));
#21866=CARTESIAN_POINT('Ctrl Pts',(3.76001591476243,1.34606837492147,0.9));
#21867=CARTESIAN_POINT('Ctrl Pts',(3.76072193310095,1.3438931143256,0.94150644476122));
#21868=CARTESIAN_POINT('Ctrl Pts',(3.76142795143945,1.34171785372973,0.98301288952244));
#21869=CARTESIAN_POINT('Ctrl Pts',(3.76213396977796,1.33954259313386,1.02451933428366));
#21870=CARTESIAN_POINT('Ctrl Pts',(7.03591386519191,1.25287427294368,0.9));
#21871=CARTESIAN_POINT('Ctrl Pts',(7.03520959909601,1.25069901234781,0.94150644476122));
#21872=CARTESIAN_POINT('Ctrl Pts',(7.03450533300011,1.24852375175194,0.98301288952244));
#21873=CARTESIAN_POINT('Ctrl Pts',(7.03380106690421,1.24634849115607,1.02451933428366));
#21874=CARTESIAN_POINT('Ctrl Pts',(10.3118118156214,1.06114656258054,0.9));
#21875=CARTESIAN_POINT('Ctrl Pts',(10.3096972650911,1.05897130198467,0.94150644476122));
#21876=CARTESIAN_POINT('Ctrl Pts',(10.3075827145608,1.0567960413888,0.98301288952244));
#21877=CARTESIAN_POINT('Ctrl Pts',(10.3054681640305,1.05462078079293,1.02451933428366));
#21878=CARTESIAN_POINT('',(10.3118118156214,1.06114656258054,0.9));
#21879=CARTESIAN_POINT('Ctrl Pts',(10.3118118156214,1.06114656258054,0.9));
#21880=CARTESIAN_POINT('Ctrl Pts',(10.3096420485163,1.05897642099582,0.941472370325488));
#21881=CARTESIAN_POINT('Ctrl Pts',(10.3074722860834,1.05680628338526,0.982944741084089));
#21882=CARTESIAN_POINT('Ctrl Pts',(10.3053025283406,1.05463614976313,1.02441711227738));
#21883=CARTESIAN_POINT('Ctrl Pts',(0.484117964332956,1.06481006947648,0.9));
#21884=CARTESIAN_POINT('Ctrl Pts',(3.76001591476244,1.34606837492147,0.9));
#21885=CARTESIAN_POINT('Ctrl Pts',(7.03591386519191,1.25287427294368,0.9));
#21886=CARTESIAN_POINT('Ctrl Pts',(10.3118118156214,1.06114656258054,0.9));
#21887=CARTESIAN_POINT('Ctrl Pts',(10.3119584735067,1.0612932457764,0.897196819041737));
#21888=CARTESIAN_POINT('Ctrl Pts',(10.3097363069231,1.05907069570186,0.939670735378922));
#21889=CARTESIAN_POINT('Ctrl Pts',(10.3075141452397,1.0568481497954,0.982144652170355));
#21890=CARTESIAN_POINT('Ctrl Pts',(10.3052919884757,1.05462560807237,1.02461856941773));
#21891=CARTESIAN_POINT('Ctrl Pts',(10.3549577591382,1.05865952187103,0.899312513938921));
#21892=CARTESIAN_POINT('Ctrl Pts',(10.3527348026837,1.05643589667682,0.941786332790264));
#21893=CARTESIAN_POINT('Ctrl Pts',(10.3505118643323,1.05421236578444,0.984260157591605));
#21894=CARTESIAN_POINT('Ctrl Pts',(10.348288915563,1.05198874626302,1.02673397710222));
#21895=CARTESIAN_POINT('Ctrl Pts',(10.427476572305,1.0195555601276,0.90106705940868));
#21896=CARTESIAN_POINT('Ctrl Pts',(10.4252515051274,1.01733143721131,0.943540744474557));
#21897=CARTESIAN_POINT('Ctrl Pts',(10.423026434404,1.01510729429004,0.986014428272043));
#21898=CARTESIAN_POINT('Ctrl Pts',(10.4208013694594,1.01288317591826,1.02848811366363));
#21899=CARTESIAN_POINT('Ctrl Pts',(10.452914163627,0.944082648463888,0.89845127988914));
#21900=CARTESIAN_POINT('Ctrl Pts',(10.4506882024692,0.941859792143813,0.940924989850352));
#21901=CARTESIAN_POINT('Ctrl Pts',(10.4484622663099,0.939636927142988,0.983398700650476));
#21902=CARTESIAN_POINT('Ctrl Pts',(10.4462363051112,0.937414078664829,1.02587241101113));
#21903=CARTESIAN_POINT('Ctrl Pts',(10.453002503567,0.911777874403687,0.896765653419433));
#21904=CARTESIAN_POINT('Ctrl Pts',(10.4507765491346,0.909555555737009,0.939239394205133));
#21905=CARTESIAN_POINT('Ctrl Pts',(10.4485505946895,0.90733324168256,0.981713135231494));
#21906=CARTESIAN_POINT('Ctrl Pts',(10.4463246402318,0.905110932257975,1.02418687649944));
#21907=CARTESIAN_POINT('',(10.4528329986453,0.911608646352005,0.9));
#21908=CARTESIAN_POINT('Ctrl Pts',(10.4463246402318,0.905110932257975,1.02418687649944));
#21909=CARTESIAN_POINT('Ctrl Pts',(10.4484940930483,0.90727683256362,0.982791250770435));
#21910=CARTESIAN_POINT('Ctrl Pts',(10.4506635458528,0.909442737267073,0.941395625270907));
#21911=CARTESIAN_POINT('Ctrl Pts',(10.4528329986453,0.911608646352005,0.9));
#21912=CARTESIAN_POINT('Ctrl Pts',(10.4528329986453,0.911608646352005,0.9));
#21913=CARTESIAN_POINT('Ctrl Pts',(10.4528329984504,0.922365992175136,0.899999999995018));
#21914=CARTESIAN_POINT('Ctrl Pts',(10.4516419184466,0.933071221555305,0.899998396191737));
#21915=CARTESIAN_POINT('Ctrl Pts',(10.4493455883239,0.943542152407774,0.899997878793429));
#21916=CARTESIAN_POINT('Ctrl Pts',(10.4474685729764,0.952101068966945,0.899997455873155));
#21917=CARTESIAN_POINT('Ctrl Pts',(10.4448518647823,0.96050416098414,0.899997731911133));
#21918=CARTESIAN_POINT('Ctrl Pts',(10.4415172538375,0.968646108261598,0.899998556768105));
#21919=CARTESIAN_POINT('Ctrl Pts',(10.4374420364703,0.978596355981088,0.899999564823172));
#21920=CARTESIAN_POINT('Ctrl Pts',(10.4323389624922,0.988051909949456,0.900001510869465));
#21921=CARTESIAN_POINT('Ctrl Pts',(10.4262707314398,0.996829854811629,0.900000879982417));
#21922=CARTESIAN_POINT('Ctrl Pts',(10.4250393574459,0.998611087749148,0.900000751961929));
#21923=CARTESIAN_POINT('Ctrl Pts',(10.4237680854757,1.0003643483506,0.900000505994341));
#21924=CARTESIAN_POINT('Ctrl Pts',(10.4224572101159,1.00208797543426,0.90000009374416));
#21925=CARTESIAN_POINT('Ctrl Pts',(10.4185057422955,1.00728363107359,0.899998851068177));
#21926=CARTESIAN_POINT('Ctrl Pts',(10.4141947510749,1.0122104380758,0.899996136506224));
#21927=CARTESIAN_POINT('Ctrl Pts',(10.4095592300387,1.01684760353016,0.899993329936423));
#21928=CARTESIAN_POINT('Ctrl Pts',(10.4019420261375,1.02446750958049,0.899988718110854));
#21929=CARTESIAN_POINT('Ctrl Pts',(10.3935294957569,1.03122853977634,0.899984126639313));
#21930=CARTESIAN_POINT('Ctrl Pts',(10.3844977038391,1.03705893037027,0.899982514537369));
#21931=CARTESIAN_POINT('Ctrl Pts',(10.3781912117148,1.04113002863034,0.899981388879436));
#21932=CARTESIAN_POINT('Ctrl Pts',(10.3715817027072,1.04474676663118,0.899981626398985));
#21933=CARTESIAN_POINT('Ctrl Pts',(10.364720849853,1.04787222446317,0.899983147799038));
#21934=CARTESIAN_POINT('Ctrl Pts',(10.3549611185069,1.05231826483487,0.899985312027903));
#21935=CARTESIAN_POINT('Ctrl Pts',(10.34479058664,1.05572789097839,0.899990169054599));
#21936=CARTESIAN_POINT('Ctrl Pts',(10.3343672593286,1.0580160164031,0.899994394012168));
#21937=CARTESIAN_POINT('Ctrl Pts',(10.3269595157814,1.05964216185967,0.899997396642827));
#21938=CARTESIAN_POINT('Ctrl Pts',(10.3194233385871,1.06070108442786,0.899999999979614));
#21939=CARTESIAN_POINT('Ctrl Pts',(10.3118118156214,1.06114656258054,0.9));
#21940=CARTESIAN_POINT('Origin',(5.4,6.06940689584926E-17,1.1));
#21941=CARTESIAN_POINT('Origin',(10.4528329986453,1.05283299864526,0.9));
#21942=CARTESIAN_POINT('',(10.4528329986453,-0.911608646352005,0.9));
#21943=CARTESIAN_POINT('Ctrl Pts',(10.4528329986453,-0.911608646352005,
0.9));
#21944=CARTESIAN_POINT('Ctrl Pts',(10.4506635458528,-0.909442737267073,
0.941395625270908));
#21945=CARTESIAN_POINT('Ctrl Pts',(10.4484940930483,-0.907276832563621,
0.982791250770435));
#21946=CARTESIAN_POINT('Ctrl Pts',(10.4463246402318,-0.905110932257975,
1.02418687649944));
#21947=CARTESIAN_POINT('',(10.4528329986453,1.05283299864526,0.9));
#21948=CARTESIAN_POINT('Ctrl Pts',(0.483981659460312,-1.06494641796617,
0.897392794396587));
#21949=CARTESIAN_POINT('Ctrl Pts',(0.486202123526484,-1.0627252433871,0.939865274484676));
#21950=CARTESIAN_POINT('Ctrl Pts',(0.488422580760962,-1.06050407431064,
0.982337755190696));
#21951=CARTESIAN_POINT('Ctrl Pts',(0.49064303113777,-1.05828291075608,1.02481023651688));
#21952=CARTESIAN_POINT('Ctrl Pts',(0.441839113682364,-1.06121395205434,
0.899406236555586));
#21953=CARTESIAN_POINT('Ctrl Pts',(0.444060746976072,-1.05899130022525,
0.941878578466898));
#21954=CARTESIAN_POINT('Ctrl Pts',(0.446282352620465,-1.05676877539366,
0.984350928552248));
#21955=CARTESIAN_POINT('Ctrl Pts',(0.448503975350841,-1.05454613107877,
1.02682327135645));
#21956=CARTESIAN_POINT('Ctrl Pts',(0.371552730979752,-1.02159229167772,
0.901018138383736));
#21957=CARTESIAN_POINT('Ctrl Pts',(0.373777362914204,-1.01936901231721,
0.943490294374253));
#21958=CARTESIAN_POINT('Ctrl Pts',(0.376002007910301,-1.01714569791452,
0.985962447794501));
#21959=CARTESIAN_POINT('Ctrl Pts',(0.378226636819208,-1.01492242480963,
1.02843460423251));
#21960=CARTESIAN_POINT('Ctrl Pts',(0.347084422593647,-0.947458158036175,
0.898424303372123));
#21961=CARTESIAN_POINT('Ctrl Pts',(0.349310306978605,-0.945236691937326,
0.940896495998714));
#21962=CARTESIAN_POINT('Ctrl Pts',(0.351536158132471,-0.943015214174121,
0.983368689735046));
#21963=CARTESIAN_POINT('Ctrl Pts',(0.353762042571371,-0.940793758946387,
1.02584088291578));
#21964=CARTESIAN_POINT('Ctrl Pts',(0.346997732921341,-0.915734826946278,
0.896770165885443));
#21965=CARTESIAN_POINT('Ctrl Pts',(0.349223608519429,-0.913514130802309,
0.939242402422435));
#21966=CARTESIAN_POINT('Ctrl Pts',(0.351449484135016,-0.911293441062403,
0.981714639293352));
#21967=CARTESIAN_POINT('Ctrl Pts',(0.35367535976817,-0.909072757750428,
1.02418687649944));
#21968=CARTESIAN_POINT('',(0.484117964332957,-1.06481006947648,0.9));
#21969=CARTESIAN_POINT('Ctrl Pts',(0.347167001354737,-0.915565952400859,
0.9));
#21970=CARTESIAN_POINT('Ctrl Pts',(0.347167001618251,-0.926324952789844,
0.899999999993398));
#21971=CARTESIAN_POINT('Ctrl Pts',(0.348355267190738,-0.937032860435638,
0.899998616841383));
#21972=CARTESIAN_POINT('Ctrl Pts',(0.350648507770679,-0.947506517879914,
0.899998360166273));
#21973=CARTESIAN_POINT('Ctrl Pts',(0.352522341068278,-0.956064664041459,
0.899998150434084));
#21974=CARTESIAN_POINT('Ctrl Pts',(0.355135157141203,-0.964467130383873,
0.899998666502847));
#21975=CARTESIAN_POINT('Ctrl Pts',(0.358466575399326,-0.972608174091076,
0.89999965996049));
#21976=CARTESIAN_POINT('Ctrl Pts',(0.362538734686669,-0.982559379305286,
0.900000874313493));
#21977=CARTESIAN_POINT('Ctrl Pts',(0.367640276064737,-0.992015301694373,
0.90000291775694));
#21978=CARTESIAN_POINT('Ctrl Pts',(0.373711018494534,-1.00079214745216,
0.900002098461893));
#21979=CARTESIAN_POINT('Ctrl Pts',(0.3746124109217,-1.00209534593109,0.900001976811805));
#21980=CARTESIAN_POINT('Ctrl Pts',(0.375535256028145,-1.00338353399439,
0.900001785555943));
#21981=CARTESIAN_POINT('Ctrl Pts',(0.376479443106529,-1.00465606108108,
0.900001505529245));
#21982=CARTESIAN_POINT('Ctrl Pts',(0.380715143239362,-1.01036472123275,
0.900000249306668));
#21983=CARTESIAN_POINT('Ctrl Pts',(0.385379830512911,-1.01575881671377,
0.899997265714102));
#21984=CARTESIAN_POINT('Ctrl Pts',(0.390428509023093,-1.02081078987204,
0.899994288896867));
#21985=CARTESIAN_POINT('Ctrl Pts',(0.398043974952909,-1.02843122547464,
0.899989798642598));
#21986=CARTESIAN_POINT('Ctrl Pts',(0.406453848296673,-1.0351976329321,0.899985566096));
#21987=CARTESIAN_POINT('Ctrl Pts',(0.415484607049401,-1.04103374418621,
0.899984276342262));
#21988=CARTESIAN_POINT('Ctrl Pts',(0.421222938370041,-1.04474213026064,
0.899983456806));
#21989=CARTESIAN_POINT('Ctrl Pts',(0.427212893823218,-1.04807424787086,
0.899983742291921));
#21990=CARTESIAN_POINT('Ctrl Pts',(0.433415948881005,-1.05100146303553,
0.899985033489932));
#21991=CARTESIAN_POINT('Ctrl Pts',(0.443112479013355,-1.05557724541753,
0.899987051872858));
#21992=CARTESIAN_POINT('Ctrl Pts',(0.453235937005982,-1.05912207412747,
0.899991654125809));
#21993=CARTESIAN_POINT('Ctrl Pts',(0.463629957379397,-1.06154692150368,
0.899995467994069));
#21994=CARTESIAN_POINT('Ctrl Pts',(0.470358492676306,-1.06311663856929,
0.899997936889288));
#21995=CARTESIAN_POINT('Ctrl Pts',(0.477201035001208,-1.06421620326297,
0.899999999975707));
#21996=CARTESIAN_POINT('Ctrl Pts',(0.484117964332956,-1.06481006947648,
0.9));
#21997=CARTESIAN_POINT('Ctrl Pts',(0.484117964332956,-1.06481006947648,
0.9));
#21998=CARTESIAN_POINT('Ctrl Pts',(0.486287923702977,-1.06263941570101,
0.941506444170342));
#21999=CARTESIAN_POINT('Ctrl Pts',(0.488457876548035,-1.06046876718106,
0.983012888930867));
#22000=CARTESIAN_POINT('Ctrl Pts',(0.490627822843887,-1.05829812393464,
1.02451933428366));
#22001=CARTESIAN_POINT('Ctrl Pts',(10.453005262311,-0.911780628641665,0.896713013448579));
#22002=CARTESIAN_POINT('Ctrl Pts',(10.4507783882972,-0.90955739189185,0.939204300891032));
#22003=CARTESIAN_POINT('Ctrl Pts',(10.4485515142709,-0.907334159758067,
0.981695588574343));
#22004=CARTESIAN_POINT('Ctrl Pts',(10.4463246402318,-0.905110932257975,
1.02418687649944));
#22005=CARTESIAN_POINT('Ctrl Pts',(10.4528874757217,-0.954853661617318,
0.898960515458773));
#22006=CARTESIAN_POINT('Ctrl Pts',(10.4506605772126,-0.952629688741643,
0.941451759962203));
#22007=CARTESIAN_POINT('Ctrl Pts',(10.4484337586651,-0.950405759674028,
0.983943010977281));
#22008=CARTESIAN_POINT('Ctrl Pts',(10.4462068600709,-0.948181794133781,
1.02643425584837));
#22009=CARTESIAN_POINT('Ctrl Pts',(10.4180804799687,-1.02952167699519,0.901043151378082));
#22010=CARTESIAN_POINT('Ctrl Pts',(10.4158548456208,-1.02729651565793,0.943534394542847));
#22011=CARTESIAN_POINT('Ctrl Pts',(10.413629193759,-1.02507134540722,0.986025636297673));
#22012=CARTESIAN_POINT('Ctrl Pts',(10.4114035625395,-1.02284618829514,1.02851687981561));
#22013=CARTESIAN_POINT('Ctrl Pts',(10.3442106925096,-1.05932070834318,0.898730950115076));
#22014=CARTESIAN_POINT('Ctrl Pts',(10.3419870251366,-1.05709644901815,0.941222341385074));
#22015=CARTESIAN_POINT('Ctrl Pts',(10.3397633429135,-1.0548722146549,0.983713733185165));
#22016=CARTESIAN_POINT('Ctrl Pts',(10.3375396837912,-1.05264796171536,1.0262051251811));
#22017=CARTESIAN_POINT('Ctrl Pts',(10.3119612275562,-1.06129600030118,0.897144178853313));
#22018=CARTESIAN_POINT('Ctrl Pts',(10.309738142952,-1.05907253204827,0.939635641919599));
#22019=CARTESIAN_POINT('Ctrl Pts',(10.3075150632522,-1.05684906796687,0.982127105440503));
#22020=CARTESIAN_POINT('Ctrl Pts',(10.3052919884757,-1.05462560807237,1.02461856941773));
#22021=CARTESIAN_POINT('',(10.3118118156214,-1.06114656258054,0.9));
#22022=CARTESIAN_POINT('Ctrl Pts',(10.3053025283406,-1.05463614976313,1.02441711227736));
#22023=CARTESIAN_POINT('Ctrl Pts',(10.3074722860834,-1.05680628338526,0.982944741084074));
#22024=CARTESIAN_POINT('Ctrl Pts',(10.3096420485163,-1.05897642099582,0.941472370325483));
#22025=CARTESIAN_POINT('Ctrl Pts',(10.3118118156214,-1.06114656258054,0.900000000000001));
#22026=CARTESIAN_POINT('Ctrl Pts',(10.3118118156214,-1.06114656258054,0.900000000000001));
#22027=CARTESIAN_POINT('Ctrl Pts',(10.322549369014,-1.06051812817027,0.899999999998837));
#22028=CARTESIAN_POINT('Ctrl Pts',(10.3331651969327,-1.05870347076406,0.899998279675625));
#22029=CARTESIAN_POINT('Ctrl Pts',(10.3434824690201,-1.05579899810317,0.899997678781422));
#22030=CARTESIAN_POINT('Ctrl Pts',(10.3519099591122,-1.05342652848477,0.899997187951103));
#22031=CARTESIAN_POINT('Ctrl Pts',(10.3601388923794,-1.05032564389788,0.899997411230107));
#22032=CARTESIAN_POINT('Ctrl Pts',(10.368065652211,-1.04652424300033,0.899998227267474));
#22033=CARTESIAN_POINT('Ctrl Pts',(10.3777613500057,-1.04187452040475,0.89999922541197));
#22034=CARTESIAN_POINT('Ctrl Pts',(10.3869029298231,-1.0362271920453,0.900001226887481));
#22035=CARTESIAN_POINT('Ctrl Pts',(10.3953114913929,-1.02965576012812,0.900000692598515));
#22036=CARTESIAN_POINT('Ctrl Pts',(10.3970212347867,-1.0283195669856,0.900000583959597));
#22037=CARTESIAN_POINT('Ctrl Pts',(10.3987005924826,-1.02694501523934,0.900000358370781));
#22038=CARTESIAN_POINT('Ctrl Pts',(10.4003479139729,-1.02553250004787,0.899999966744969));
#22039=CARTESIAN_POINT('Ctrl Pts',(10.4052955867552,-1.02129005981461,0.899998790510468));
#22040=CARTESIAN_POINT('Ctrl Pts',(10.4099546972526,-1.01670546321193,0.899996154952331));
#22041=CARTESIAN_POINT('Ctrl Pts',(10.4143066574475,-1.01181472964029,0.899993423989004));
#22042=CARTESIAN_POINT('Ctrl Pts',(10.4214686344271,-1.00376609875091,0.899988929670213));
#22043=CARTESIAN_POINT('Ctrl Pts',(10.4277268376922,-0.994973664259555,
0.899984438878373));
#22044=CARTESIAN_POINT('Ctrl Pts',(10.4330201329469,-0.98561748607337,0.899982870029797));
#22045=CARTESIAN_POINT('Ctrl Pts',(10.4367196060238,-0.979078472540648,
0.89998177356478));
#22046=CARTESIAN_POINT('Ctrl Pts',(10.4399470827666,-0.972263038755176,
0.89998201356482));
#22047=CARTESIAN_POINT('Ctrl Pts',(10.4426687152005,-0.965225084739993,
0.899983510148066));
#22048=CARTESIAN_POINT('Ctrl Pts',(10.4465375225522,-0.955220615401818,
0.899985637544916));
#22049=CARTESIAN_POINT('Ctrl Pts',(10.4493477346146,-0.944866529467853,
0.899990392295554));
#22050=CARTESIAN_POINT('Ctrl Pts',(10.4510237312406,-0.934325606572895,
0.899994522211612));
#22051=CARTESIAN_POINT('Ctrl Pts',(10.452215546318,-0.926829869027477,0.899997459029114));
#22052=CARTESIAN_POINT('Ctrl Pts',(10.452832998309,-0.919238945488459,0.899999999973399));
#22053=CARTESIAN_POINT('Ctrl Pts',(10.4528329986453,-0.911608646352005,
0.9));
#22054=CARTESIAN_POINT('Origin',(5.4,0.,0.9));
#22055=CARTESIAN_POINT('Ctrl Pts',(10.3118118156214,-1.06114656258054,0.9));
#22056=CARTESIAN_POINT('Ctrl Pts',(7.03591386519191,-1.25287427294368,0.9));
#22057=CARTESIAN_POINT('Ctrl Pts',(3.76001591476243,-1.34606837492147,0.9));
#22058=CARTESIAN_POINT('Ctrl Pts',(0.484117964332957,-1.06481006947648,
0.9));
#22059=CARTESIAN_POINT('Ctrl Pts',(10.3118118156214,-1.06114656258054,0.9));
#22060=CARTESIAN_POINT('Ctrl Pts',(10.3096972650911,-1.05897130198467,0.94150644476122));
#22061=CARTESIAN_POINT('Ctrl Pts',(10.3075827145608,-1.0567960413888,0.98301288952244));
#22062=CARTESIAN_POINT('Ctrl Pts',(10.3054681640305,-1.05462078079293,1.02451933428366));
#22063=CARTESIAN_POINT('Ctrl Pts',(7.03591386519191,-1.25287427294368,0.9));
#22064=CARTESIAN_POINT('Ctrl Pts',(7.03520959909601,-1.25069901234781,0.94150644476122));
#22065=CARTESIAN_POINT('Ctrl Pts',(7.03450533300011,-1.24852375175194,0.98301288952244));
#22066=CARTESIAN_POINT('Ctrl Pts',(7.03380106690421,-1.24634849115607,1.02451933428366));
#22067=CARTESIAN_POINT('Ctrl Pts',(3.76001591476244,-1.34606837492147,0.9));
#22068=CARTESIAN_POINT('Ctrl Pts',(3.76072193310095,-1.3438931143256,0.94150644476122));
#22069=CARTESIAN_POINT('Ctrl Pts',(3.76142795143946,-1.34171785372973,0.98301288952244));
#22070=CARTESIAN_POINT('Ctrl Pts',(3.76213396977796,-1.33954259313386,1.02451933428366));
#22071=CARTESIAN_POINT('Ctrl Pts',(0.484117964332957,-1.06481006947648,
0.9));
#22072=CARTESIAN_POINT('Ctrl Pts',(0.486234267105876,-1.06263480888061,
0.94150644476122));
#22073=CARTESIAN_POINT('Ctrl Pts',(0.488350569878795,-1.06045954828474,
0.98301288952244));
#22074=CARTESIAN_POINT('Ctrl Pts',(0.490466872651714,-1.05828428768887,
1.02451933428366));
#22115=UNCERTAINTY_MEASURE_WITH_UNIT(LENGTH_MEASURE(0.001),#22130,
'DISTANCE_ACCURACY_VALUE',
'Maximum model space distance between geometric entities at asserted c
onnectivities');
#22117=UNCERTAINTY_MEASURE_WITH_UNIT(LENGTH_MEASURE(0.001),#22130,
'DISTANCE_ACCURACY_VALUE',
'Maximum model space distance between geometric entities at asserted c
onnectivities');
#22127=(
GEOMETRIC_REPRESENTATION_CONTEXT(3)
GLOBAL_UNCERTAINTY_ASSIGNED_CONTEXT((#22115))
GLOBAL_UNIT_ASSIGNED_CONTEXT((#22130,#22132,#22133))
REPRESENTATION_CONTEXT('','3D')
);
#22129=(
GEOMETRIC_REPRESENTATION_CONTEXT(3)
GLOBAL_UNCERTAINTY_ASSIGNED_CONTEXT((#22117))
GLOBAL_UNIT_ASSIGNED_CONTEXT((#22130,#22132,#22133))
REPRESENTATION_CONTEXT('','3D')
);
#22130=(
LENGTH_UNIT()
NAMED_UNIT(*)
SI_UNIT(.CENTI.,.METRE.)
);
#22132=(
NAMED_UNIT(*)
PLANE_ANGLE_UNIT()
SI_UNIT($,.RADIAN.)
);
#22133=(
NAMED_UNIT(*)
SI_UNIT($,.STERADIAN.)
SOLID_ANGLE_UNIT()
);
#22143=SHAPE_DEFINITION_REPRESENTATION(#22154,#22181);
#22154=PRODUCT_DEFINITION_SHAPE('',$,#22193);
#22181=SHAPE_REPRESENTATION('',(#9422),#22127);
#22183=PRODUCT_DEFINITION_CONTEXT('part definition',#22218,'design');
#22193=PRODUCT_DEFINITION('2026-11-10-05-10-49-242','Soft grip layer',#22204,
#22183);
#22204=PRODUCT_DEFINITION_FORMATION('',$,#22229);
#22218=APPLICATION_CONTEXT(
'Core Data for Automotive Mechanical Design Process');
#22219=PRODUCT_CONTEXT('part definition',#22218,'mechanical');
#22229=PRODUCT('2026-11-10-05-10-49-242','Soft grip layer',$,(#22219));
#22237=PRESENTATION_STYLE_ASSIGNMENT((#22245));
#22245=SURFACE_STYLE_USAGE(.BOTH.,#22253);
#22253=SURFACE_SIDE_STYLE('',(#22261));
#22261=SURFACE_STYLE_FILL_AREA(#22269);
#22269=FILL_AREA_STYLE('Sky blue soft grip',(#22277));
#22277=FILL_AREA_STYLE_COLOUR('Sky blue soft grip',#22285);
#22285=COLOUR_RGB('Sky blue soft grip',0.317647058823529,0.686274509803922,
0.890196078431372);
ENDSEC;
END-ISO-10303-21;
